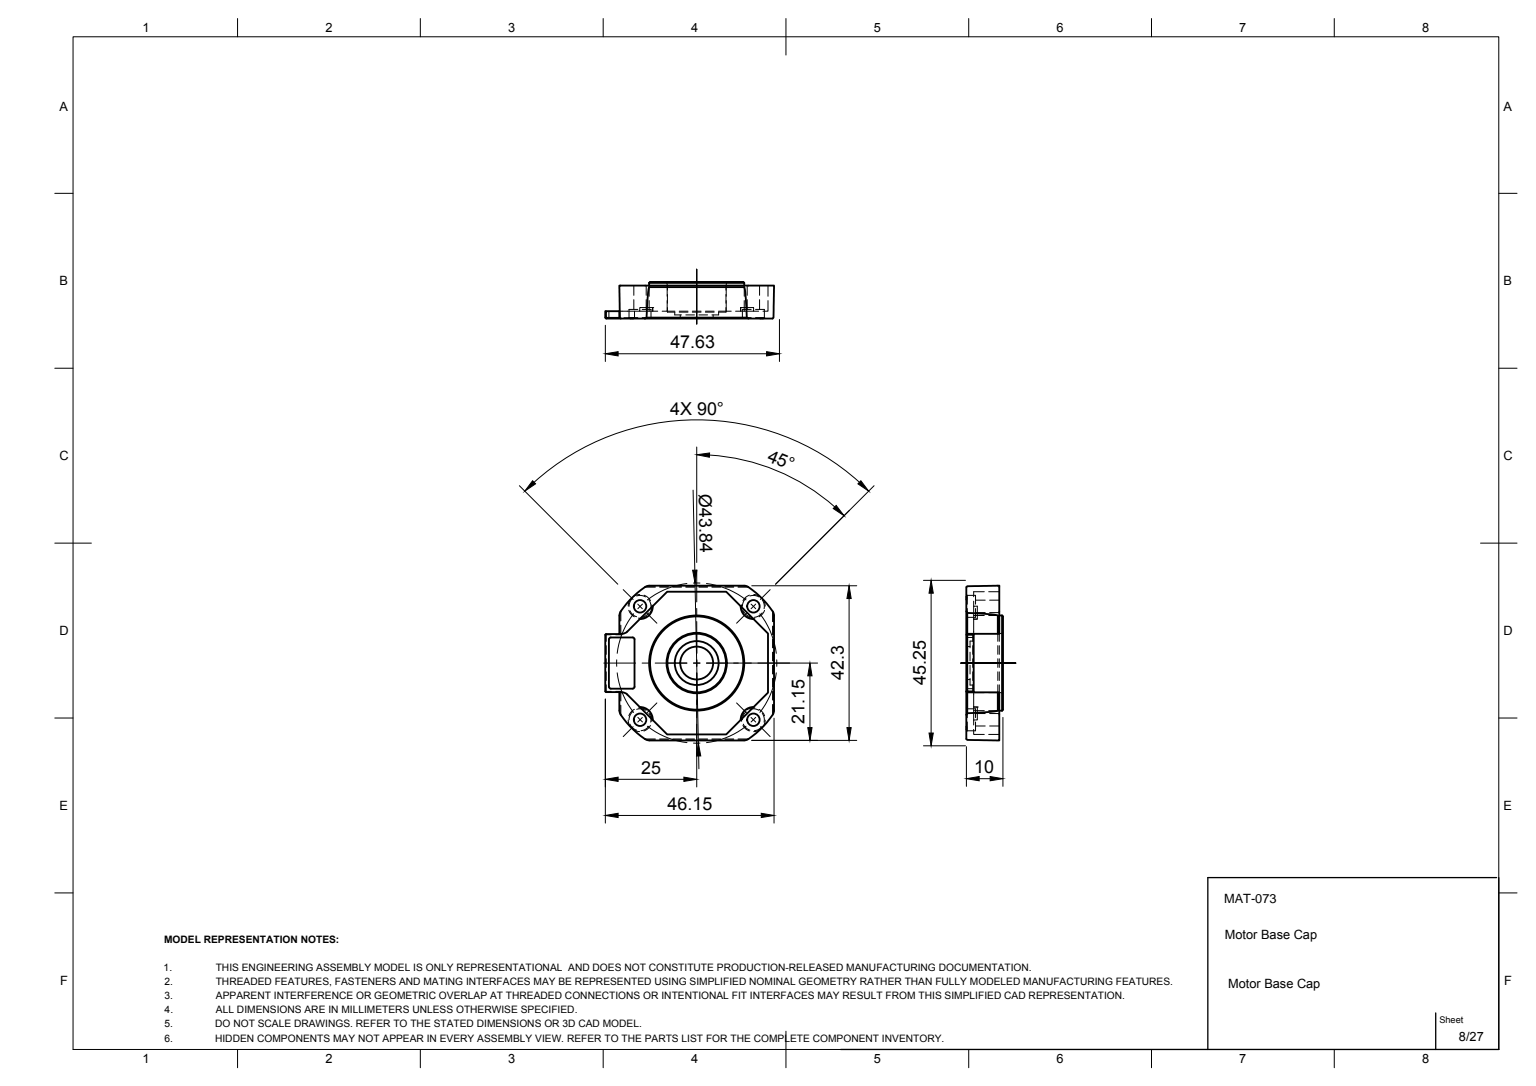
ISO-10303-21;
HEADER;
/* Generated by software containing ST-Developer
 * from STEP Tools, Inc. (www.steptools.com) 
 */

FILE_DESCRIPTION(
/* description */ ('CAx-IF Rec.Pracs.---Representation and Presentation of Product Manufa
cturing Information (PMI)---4.0---2014-10-13'),
/* implementation_level */ '2;1');

FILE_NAME(
/* name */ 'Motor Base Cap.step',
/* time_stamp */ '2026-10-24T18:52:33-07:00',
/* author */ (''),
/* organization */ (''),
/* preprocessor_version */ 'ST-DEVELOPER v20.2',
/* originating_system */ 'Autodesk Translation Framework v15.17.0.0',
/* authorisation */ '');

FILE_SCHEMA (('AP242_MANAGED_MODEL_BASED_3D_ENGINEERING_MIM_LF { 1 0 10303 442 2 1 4 }'));
ENDSEC;

DATA;
#10=MECHANICAL_DESIGN_GEOMETRIC_PRESENTATION_REPRESENTATION('',(#419),#34876);
#174=CONICAL_SURFACE('',#20658,0.003125,0.785398163397447);
#175=CONICAL_SURFACE('',#20665,0.003125,0.785398163397447);
#176=CONICAL_SURFACE('',#20672,0.003125,0.785398163397447);
#177=CONICAL_SURFACE('',#20689,0.003125,0.785398163397447);
#178=CONICAL_SURFACE('',#20758,0.012875,0.785398163397446);
#179=CONICAL_SURFACE('',#20765,0.008125,0.244978663126864);
#216=B_SPLINE_CURVE_WITH_KNOTS('',3,(#30332,#30333,#30334,#30335,#30336,
#30337),.UNSPECIFIED.,.F.,.F.,(4,2,4),(1.58777834959488,1.67090244580867,
1.70100758687363),.UNSPECIFIED.);
#217=B_SPLINE_CURVE_WITH_KNOTS('',3,(#30373,#30374,#30375,#30376,#30377,
#30378),.UNSPECIFIED.,.F.,.F.,(4,2,4),(1.58777834958732,1.67090244580931,
1.70100758688213),.UNSPECIFIED.);
#218=B_SPLINE_CURVE_WITH_KNOTS('',3,(#30414,#30415,#30416,#30417,#30418,
#30419),.UNSPECIFIED.,.F.,.F.,(4,2,4),(1.58777834957897,1.67090244581023,
1.70100758689154),.UNSPECIFIED.);
#219=B_SPLINE_CURVE_WITH_KNOTS('',3,(#30471,#30472,#30473,#30474,#30475,
#30476),.UNSPECIFIED.,.F.,.F.,(4,2,4),(1.58777834959617,1.67090244580851,
1.70100758687202),.UNSPECIFIED.);
#300=ELLIPSE('',#20594,0.114597376996511,0.00199999999998973);
#301=ELLIPSE('',#20596,0.00280406412973375,0.00199999999998973);
#302=ELLIPSE('',#20598,0.0352260556299788,0.0251250000000126);
#303=ELLIPSE('',#20600,0.0352260556299788,0.0251250000000126);
#304=ELLIPSE('',#20604,0.00280406412976774,0.00200000000001397);
#305=ELLIPSE('',#20606,0.114597376997899,0.00200000000001397);
#306=ELLIPSE('',#20609,0.114597376996524,0.00199999999998997);
#307=ELLIPSE('',#20611,0.00280406412973409,0.00199999999998997);
#308=ELLIPSE('',#20613,0.0352260556299805,0.0251250000000138);
#309=ELLIPSE('',#20615,0.0352260556299805,0.0251250000000138);
#310=ELLIPSE('',#20619,0.00280406412974482,0.00199999999999762);
#311=ELLIPSE('',#20621,0.114597376996964,0.00199999999999762);
#312=ELLIPSE('',#20624,0.114597376997842,0.00200000000001296);
#313=ELLIPSE('',#20626,0.00280406412976633,0.00200000000001296);
#314=ELLIPSE('',#20628,0.0352260556299806,0.0251250000000138);
#315=ELLIPSE('',#20630,0.0352260556299803,0.0251250000000138);
#316=ELLIPSE('',#20638,0.00280406412973409,0.00199999999998998);
#317=ELLIPSE('',#20639,0.114597376996526,0.00199999999998998);
#318=ELLIPSE('',#20642,0.0352260556300019,0.0251250000000291);
#319=ELLIPSE('',#20645,0.0352260556300016,0.0251250000000291);
#320=ELLIPSE('',#20648,0.114597376997269,0.00200000000000295);
#321=ELLIPSE('',#20649,0.00280406412975229,0.00200000000000295);
#322=ELLIPSE('',#20653,0.114597376996301,0.00199999999998605);
#323=ELLIPSE('',#20654,0.00280406412972858,0.00199999999998605);
#353=SHAPE_REPRESENTATION_RELATIONSHIP('SRR','None',#34990,#386);
#386=ADVANCED_BREP_SHAPE_REPRESENTATION('',(#452),#34848);
#419=STYLED_ITEM('',(#35159),#452);
#452=MANIFOLD_SOLID_BREP('Motor Base Cap',#19559);
#503=FACE_BOUND('',#6175,.T.);
#504=FACE_BOUND('',#6184,.T.);
#505=FACE_BOUND('',#6185,.T.);
#506=FACE_BOUND('',#6186,.T.);
#507=FACE_BOUND('',#6187,.T.);
#508=FACE_BOUND('',#6224,.T.);
#509=FACE_BOUND('',#6229,.T.);
#510=FACE_BOUND('',#6232,.T.);
#511=FACE_BOUND('',#6235,.T.);
#512=FACE_BOUND('',#6238,.T.);
#513=FACE_BOUND('',#6241,.T.);
#514=FACE_BOUND('',#6242,.T.);
#515=FACE_BOUND('',#6245,.T.);
#516=FACE_BOUND('',#6247,.T.);
#719=PLANE('',#20592);
#720=PLANE('',#20607);
#721=PLANE('',#20622);
#722=PLANE('',#20633);
#723=PLANE('',#20634);
#724=PLANE('',#20635);
#725=PLANE('',#20636);
#726=PLANE('',#20655);
#727=PLANE('',#20656);
#728=PLANE('',#20657);
#729=PLANE('',#20663);
#730=PLANE('',#20664);
#731=PLANE('',#20670);
#732=PLANE('',#20671);
#733=PLANE('',#20677);
#734=PLANE('',#20678);
#735=PLANE('',#20679);
#736=PLANE('',#20680);
#737=PLANE('',#20681);
#738=PLANE('',#20699);
#739=PLANE('',#20700);
#740=PLANE('',#20708);
#741=PLANE('',#20709);
#742=PLANE('',#20710);
#743=PLANE('',#20711);
#744=PLANE('',#20712);
#745=PLANE('',#20713);
#746=PLANE('',#20714);
#747=PLANE('',#20718);
#748=PLANE('',#20722);
#749=PLANE('',#20726);
#750=PLANE('',#20730);
#751=PLANE('',#20731);
#752=PLANE('',#20732);
#753=PLANE('',#20733);
#754=PLANE('',#20736);
#755=PLANE('',#20737);
#756=PLANE('',#20741);
#757=PLANE('',#20745);
#758=PLANE('',#20749);
#759=PLANE('',#20750);
#760=PLANE('',#20751);
#761=PLANE('',#20755);
#762=PLANE('',#20756);
#763=PLANE('',#20757);
#764=PLANE('',#20761);
#765=PLANE('',#20770);
#766=PLANE('',#20773);
#767=PLANE('',#20776);
#768=PLANE('',#20779);
#769=PLANE('',#20782);
#770=PLANE('',#20786);
#771=PLANE('',#20787);
#772=PLANE('',#20788);
#773=PLANE('',#20789);
#774=PLANE('',#20790);
#775=PLANE('',#20791);
#1478=LINE('',#30306,#3077);
#1479=LINE('',#30308,#3078);
#1480=LINE('',#30310,#3079);
#1481=LINE('',#30311,#3080);
#1482=LINE('',#30318,#3081);
#1483=LINE('',#30326,#3082);
#1484=LINE('',#30345,#3083);
#1485=LINE('',#30349,#3084);
#1486=LINE('',#30351,#3085);
#1487=LINE('',#30352,#3086);
#1488=LINE('',#30359,#3087);
#1489=LINE('',#30367,#3088);
#1490=LINE('',#30386,#3089);
#1491=LINE('',#30390,#3090);
#1492=LINE('',#30392,#3091);
#1493=LINE('',#30393,#3092);
#1494=LINE('',#30400,#3093);
#1495=LINE('',#30408,#3094);
#1496=LINE('',#30424,#3095);
#1497=LINE('',#30426,#3096);
#1498=LINE('',#30428,#3097);
#1499=LINE('',#30429,#3098);
#1500=LINE('',#30433,#3099);
#1501=LINE('',#30435,#3100);
#1502=LINE('',#30437,#3101);
#1503=LINE('',#30438,#3102);
#1504=LINE('',#30441,#3103);
#1505=LINE('',#30443,#3104);
#1506=LINE('',#30445,#3105);
#1507=LINE('',#30446,#3106);
#1508=LINE('',#30450,#3107);
#1509=LINE('',#30452,#3108);
#1510=LINE('',#30454,#3109);
#1511=LINE('',#30455,#3110);
#1512=LINE('',#30463,#3111);
#1513=LINE('',#30482,#3112);
#1514=LINE('',#30492,#3113);
#1515=LINE('',#30498,#3114);
#1516=LINE('',#30500,#3115);
#1517=LINE('',#30501,#3116);
#1518=LINE('',#30504,#3117);
#1519=LINE('',#30506,#3118);
#1520=LINE('',#30508,#3119);
#1521=LINE('',#30509,#3120);
#1522=LINE('',#30511,#3121);
#1523=LINE('',#30517,#3122);
#1524=LINE('',#30522,#3123);
#1525=LINE('',#30524,#3124);
#1526=LINE('',#30530,#3125);
#1527=LINE('',#30535,#3126);
#1528=LINE('',#30537,#3127);
#1529=LINE('',#30543,#3128);
#1530=LINE('',#30549,#3129);
#1531=LINE('',#30551,#3130);
#1532=LINE('',#30552,#3131);
#1533=LINE('',#30555,#3132);
#1534=LINE('',#30557,#3133);
#1535=LINE('',#30558,#3134);
#1536=LINE('',#30561,#3135);
#1537=LINE('',#30562,#3136);
#1538=LINE('',#30563,#3137);
#1539=LINE('',#30566,#3138);
#1540=LINE('',#30568,#3139);
#1541=LINE('',#30569,#3140);
#1542=LINE('',#30571,#3141);
#1543=LINE('',#30573,#3142);
#1544=LINE('',#30575,#3143);
#1545=LINE('',#30576,#3144);
#1546=LINE('',#30585,#3145);
#1547=LINE('',#30589,#3146);
#1548=LINE('',#30594,#3147);
#1549=LINE('',#30599,#3148);
#1550=LINE('',#30603,#3149);
#1551=LINE('',#30609,#3150);
#1552=LINE('',#30612,#3151);
#1553=LINE('',#30615,#3152);
#1554=LINE('',#30616,#3153);
#1555=LINE('',#30617,#3154);
#1556=LINE('',#30620,#3155);
#1557=LINE('',#30622,#3156);
#1558=LINE('',#30624,#3157);
#1559=LINE('',#30626,#3158);
#1560=LINE('',#30628,#3159);
#1561=LINE('',#30630,#3160);
#1562=LINE('',#30632,#3161);
#1563=LINE('',#30635,#3162);
#1564=LINE('',#30646,#3163);
#1565=LINE('',#30649,#3164);
#1566=LINE('',#30652,#3165);
#1567=LINE('',#30654,#3166);
#1568=LINE('',#30656,#3167);
#1569=LINE('',#30658,#3168);
#1570=LINE('',#30660,#3169);
#1571=LINE('',#30661,#3170);
#1572=LINE('',#30663,#3171);
#1573=LINE('',#30664,#3172);
#1574=LINE('',#30666,#3173);
#1575=LINE('',#30667,#3174);
#1576=LINE('',#30670,#3175);
#1577=LINE('',#30671,#3176);
#1578=LINE('',#30674,#3177);
#1579=LINE('',#30675,#3178);
#1580=LINE('',#30677,#3179);
#1581=LINE('',#30680,#3180);
#1582=LINE('',#30682,#3181);
#1583=LINE('',#30683,#3182);
#1584=LINE('',#30689,#3183);
#1585=LINE('',#30692,#3184);
#1586=LINE('',#30695,#3185);
#1587=LINE('',#30697,#3186);
#1588=LINE('',#30698,#3187);
#1589=LINE('',#30703,#3188);
#1590=LINE('',#30707,#3189);
#1591=LINE('',#30709,#3190);
#1592=LINE('',#30710,#3191);
#1593=LINE('',#30715,#3192);
#1594=LINE('',#30719,#3193);
#1595=LINE('',#30721,#3194);
#1596=LINE('',#30722,#3195);
#1597=LINE('',#30727,#3196);
#1598=LINE('',#30730,#3197);
#1599=LINE('',#30732,#3198);
#1600=LINE('',#30735,#3199);
#1601=LINE('',#30739,#3200);
#1602=LINE('',#30741,#3201);
#1603=LINE('',#30742,#3202);
#1604=LINE('',#30744,#3203);
#1605=LINE('',#30750,#3204);
#1606=LINE('',#30753,#3205);
#1607=LINE('',#30755,#3206);
#1608=LINE('',#30765,#3207);
#1609=LINE('',#30768,#3208);
#1610=LINE('',#30770,#3209);
#1611=LINE('',#30772,#3210);
#1612=LINE('',#30774,#3211);
#1613=LINE('',#30775,#3212);
#1614=LINE('',#30778,#3213);
#1615=LINE('',#30779,#3214);
#1616=LINE('',#30781,#3215);
#1617=LINE('',#30782,#3216);
#1618=LINE('',#30788,#3217);
#1619=LINE('',#30791,#3218);
#1620=LINE('',#30793,#3219);
#1621=LINE('',#30796,#3220);
#1622=LINE('',#30797,#3221);
#1623=LINE('',#30799,#3222);
#1624=LINE('',#30800,#3223);
#1625=LINE('',#30806,#3224);
#1626=LINE('',#30814,#3225);
#1627=LINE('',#30819,#3226);
#1628=LINE('',#30823,#3227);
#1629=LINE('',#30829,#3228);
#1630=LINE('',#30834,#3229);
#1631=LINE('',#30839,#3230);
#1632=LINE('',#30844,#3231);
#1633=LINE('',#30846,#3232);
#1634=LINE('',#30847,#3233);
#1635=LINE('',#30848,#3234);
#1636=LINE('',#30853,#3235);
#3077=VECTOR('',#23937,0.01);
#3078=VECTOR('',#23938,0.01);
#3079=VECTOR('',#23939,0.01);
#3080=VECTOR('',#23940,0.01);
#3081=VECTOR('',#23947,0.01);
#3082=VECTOR('',#23956,0.01);
#3083=VECTOR('',#23969,0.01);
#3084=VECTOR('',#23974,0.01);
#3085=VECTOR('',#23975,0.01);
#3086=VECTOR('',#23976,0.01);
#3087=VECTOR('',#23983,0.01);
#3088=VECTOR('',#23992,0.01);
#3089=VECTOR('',#24005,0.01);
#3090=VECTOR('',#24010,0.01);
#3091=VECTOR('',#24011,0.01);
#3092=VECTOR('',#24012,0.01);
#3093=VECTOR('',#24019,0.01);
#3094=VECTOR('',#24028,0.01);
#3095=VECTOR('',#24037,0.01);
#3096=VECTOR('',#24038,0.01);
#3097=VECTOR('',#24039,0.01);
#3098=VECTOR('',#24040,0.01);
#3099=VECTOR('',#24043,0.01);
#3100=VECTOR('',#24044,0.01);
#3101=VECTOR('',#24045,0.01);
#3102=VECTOR('',#24046,0.01);
#3103=VECTOR('',#24049,0.01);
#3104=VECTOR('',#24050,0.01);
#3105=VECTOR('',#24051,0.01);
#3106=VECTOR('',#24052,0.01);
#3107=VECTOR('',#24055,0.01);
#3108=VECTOR('',#24056,0.01);
#3109=VECTOR('',#24057,0.01);
#3110=VECTOR('',#24058,0.01);
#3111=VECTOR('',#24067,0.01);
#3112=VECTOR('',#24080,0.01);
#3113=VECTOR('',#24093,0.01);
#3114=VECTOR('',#24100,0.01);
#3115=VECTOR('',#24101,0.01);
#3116=VECTOR('',#24102,0.01);
#3117=VECTOR('',#24105,0.01);
#3118=VECTOR('',#24106,0.01);
#3119=VECTOR('',#24107,0.01);
#3120=VECTOR('',#24108,0.01);
#3121=VECTOR('',#24111,1.);
#3122=VECTOR('',#24116,0.003125);
#3123=VECTOR('',#24125,1.);
#3124=VECTOR('',#24128,1.);
#3125=VECTOR('',#24133,0.003125);
#3126=VECTOR('',#24142,1.);
#3127=VECTOR('',#24145,1.);
#3128=VECTOR('',#24150,0.003125);
#3129=VECTOR('',#24159,1.);
#3130=VECTOR('',#24160,1.);
#3131=VECTOR('',#24161,1.);
#3132=VECTOR('',#24164,1.);
#3133=VECTOR('',#24165,1.);
#3134=VECTOR('',#24166,1.);
#3135=VECTOR('',#24169,1.);
#3136=VECTOR('',#24170,1.);
#3137=VECTOR('',#24171,1.);
#3138=VECTOR('',#24174,1.);
#3139=VECTOR('',#24175,1.);
#3140=VECTOR('',#24176,1.);
#3141=VECTOR('',#24179,1.);
#3142=VECTOR('',#24180,1.);
#3143=VECTOR('',#24181,1.);
#3144=VECTOR('',#24182,1.);
#3145=VECTOR('',#24193,0.003);
#3146=VECTOR('',#24198,0.003);
#3147=VECTOR('',#24203,0.003125);
#3148=VECTOR('',#24210,0.003);
#3149=VECTOR('',#24215,0.003);
#3150=VECTOR('',#24220,1.);
#3151=VECTOR('',#24223,1.);
#3152=VECTOR('',#24226,1.);
#3153=VECTOR('',#24227,1.);
#3154=VECTOR('',#24228,1.);
#3155=VECTOR('',#24231,1.);
#3156=VECTOR('',#24232,1.);
#3157=VECTOR('',#24233,1.);
#3158=VECTOR('',#24234,1.);
#3159=VECTOR('',#24235,1.);
#3160=VECTOR('',#24236,1.);
#3161=VECTOR('',#24237,1.);
#3162=VECTOR('',#24240,1.);
#3163=VECTOR('',#24251,1.);
#3164=VECTOR('',#24254,1.);
#3165=VECTOR('',#24257,1.);
#3166=VECTOR('',#24258,1.);
#3167=VECTOR('',#24259,1.);
#3168=VECTOR('',#24260,1.);
#3169=VECTOR('',#24261,1.);
#3170=VECTOR('',#24262,1.);
#3171=VECTOR('',#24265,1.);
#3172=VECTOR('',#24266,1.);
#3173=VECTOR('',#24269,1.);
#3174=VECTOR('',#24270,1.);
#3175=VECTOR('',#24273,1.);
#3176=VECTOR('',#24274,1.);
#3177=VECTOR('',#24277,1.);
#3178=VECTOR('',#24278,1.);
#3179=VECTOR('',#24281,1.);
#3180=VECTOR('',#24284,1.);
#3181=VECTOR('',#24285,1.);
#3182=VECTOR('',#24286,1.);
#3183=VECTOR('',#24291,1.);
#3184=VECTOR('',#24294,1.);
#3185=VECTOR('',#24297,1.);
#3186=VECTOR('',#24298,1.);
#3187=VECTOR('',#24299,1.);
#3188=VECTOR('',#24304,1.);
#3189=VECTOR('',#24309,1.);
#3190=VECTOR('',#24310,1.);
#3191=VECTOR('',#24311,1.);
#3192=VECTOR('',#24316,1.);
#3193=VECTOR('',#24321,1.);
#3194=VECTOR('',#24322,1.);
#3195=VECTOR('',#24323,1.);
#3196=VECTOR('',#24328,1.);
#3197=VECTOR('',#24333,1.);
#3198=VECTOR('',#24336,1.);
#3199=VECTOR('',#24341,1.);
#3200=VECTOR('',#24346,0.0045);
#3201=VECTOR('',#24349,1.);
#3202=VECTOR('',#24350,1.);
#3203=VECTOR('',#24353,1.);
#3204=VECTOR('',#24358,1.);
#3205=VECTOR('',#24361,1.);
#3206=VECTOR('',#24364,1.);
#3207=VECTOR('',#24377,1.);
#3208=VECTOR('',#24380,1.);
#3209=VECTOR('',#24383,1.);
#3210=VECTOR('',#24386,1.);
#3211=VECTOR('',#24387,1.);
#3212=VECTOR('',#24388,1.);
#3213=VECTOR('',#24391,1.);
#3214=VECTOR('',#24392,1.);
#3215=VECTOR('',#24393,1.);
#3216=VECTOR('',#24394,1.);
#3217=VECTOR('',#24399,1.);
#3218=VECTOR('',#24402,1.);
#3219=VECTOR('',#24405,1.);
#3220=VECTOR('',#24408,1.);
#3221=VECTOR('',#24409,1.);
#3222=VECTOR('',#24410,1.);
#3223=VECTOR('',#24411,1.);
#3224=VECTOR('',#24418,0.012875);
#3225=VECTOR('',#24429,0.013);
#3226=VECTOR('',#24434,0.008125);
#3227=VECTOR('',#24439,0.008);
#3228=VECTOR('',#24448,0.0017);
#3229=VECTOR('',#24455,0.0017);
#3230=VECTOR('',#24462,0.0017);
#3231=VECTOR('',#24469,0.0017);
#3232=VECTOR('',#24472,1.);
#3233=VECTOR('',#24473,1.);
#3234=VECTOR('',#24474,1.);
#3235=VECTOR('',#24479,0.006);
#4430=CYLINDRICAL_SURFACE('',#20593,0.00199999999998973);
#4431=CYLINDRICAL_SURFACE('',#20597,0.0251250000000126);
#4432=CYLINDRICAL_SURFACE('',#20603,0.00200000000001397);
#4433=CYLINDRICAL_SURFACE('',#20608,0.00199999999998997);
#4434=CYLINDRICAL_SURFACE('',#20612,0.0251250000000138);
#4435=CYLINDRICAL_SURFACE('',#20618,0.00199999999999762);
#4436=CYLINDRICAL_SURFACE('',#20623,0.00200000000001296);
#4437=CYLINDRICAL_SURFACE('',#20627,0.0251250000000138);
#4438=CYLINDRICAL_SURFACE('',#20637,0.00199999999998998);
#4439=CYLINDRICAL_SURFACE('',#20641,0.0251250000000291);
#4440=CYLINDRICAL_SURFACE('',#20647,0.00200000000000295);
#4441=CYLINDRICAL_SURFACE('',#20651,0.00199999999998605);
#4442=CYLINDRICAL_SURFACE('',#20685,0.003);
#4443=CYLINDRICAL_SURFACE('',#20687,0.003);
#4444=CYLINDRICAL_SURFACE('',#20692,0.003);
#4445=CYLINDRICAL_SURFACE('',#20694,0.003);
#4446=CYLINDRICAL_SURFACE('',#20696,0.002);
#4447=CYLINDRICAL_SURFACE('',#20706,0.002);
#4448=CYLINDRICAL_SURFACE('',#20715,0.0005);
#4449=CYLINDRICAL_SURFACE('',#20719,0.0005);
#4450=CYLINDRICAL_SURFACE('',#20723,0.0005);
#4451=CYLINDRICAL_SURFACE('',#20727,0.0005);
#4452=CYLINDRICAL_SURFACE('',#20734,0.0045);
#4453=CYLINDRICAL_SURFACE('',#20738,0.00347964100813058);
#4454=CYLINDRICAL_SURFACE('',#20742,0.00347964100813058);
#4455=CYLINDRICAL_SURFACE('',#20746,0.00347964100813058);
#4456=CYLINDRICAL_SURFACE('',#20752,0.00347964100813058);
#4457=CYLINDRICAL_SURFACE('',#20763,0.013);
#4458=CYLINDRICAL_SURFACE('',#20768,0.008);
#4459=CYLINDRICAL_SURFACE('',#20772,0.0017);
#4460=CYLINDRICAL_SURFACE('',#20775,0.0017);
#4461=CYLINDRICAL_SURFACE('',#20778,0.0017);
#4462=CYLINDRICAL_SURFACE('',#20781,0.0017);
#4463=CYLINDRICAL_SURFACE('',#20783,0.006);
#5073=FACE_OUTER_BOUND('',#6141,.T.);
#5074=FACE_OUTER_BOUND('',#6142,.T.);
#5075=FACE_OUTER_BOUND('',#6143,.T.);
#5076=FACE_OUTER_BOUND('',#6144,.T.);
#5077=FACE_OUTER_BOUND('',#6145,.T.);
#5078=FACE_OUTER_BOUND('',#6146,.T.);
#5079=FACE_OUTER_BOUND('',#6147,.T.);
#5080=FACE_OUTER_BOUND('',#6148,.T.);
#5081=FACE_OUTER_BOUND('',#6149,.T.);
#5082=FACE_OUTER_BOUND('',#6150,.T.);
#5083=FACE_OUTER_BOUND('',#6151,.T.);
#5084=FACE_OUTER_BOUND('',#6152,.T.);
#5085=FACE_OUTER_BOUND('',#6153,.T.);
#5086=FACE_OUTER_BOUND('',#6154,.T.);
#5087=FACE_OUTER_BOUND('',#6155,.T.);
#5088=FACE_OUTER_BOUND('',#6156,.T.);
#5089=FACE_OUTER_BOUND('',#6157,.T.);
#5090=FACE_OUTER_BOUND('',#6158,.T.);
#5091=FACE_OUTER_BOUND('',#6159,.T.);
#5092=FACE_OUTER_BOUND('',#6160,.T.);
#5093=FACE_OUTER_BOUND('',#6161,.T.);
#5094=FACE_OUTER_BOUND('',#6162,.T.);
#5095=FACE_OUTER_BOUND('',#6163,.T.);
#5096=FACE_OUTER_BOUND('',#6164,.T.);
#5097=FACE_OUTER_BOUND('',#6165,.T.);
#5098=FACE_OUTER_BOUND('',#6166,.T.);
#5099=FACE_OUTER_BOUND('',#6167,.T.);
#5100=FACE_OUTER_BOUND('',#6168,.T.);
#5101=FACE_OUTER_BOUND('',#6169,.T.);
#5102=FACE_OUTER_BOUND('',#6170,.T.);
#5103=FACE_OUTER_BOUND('',#6171,.T.);
#5104=FACE_OUTER_BOUND('',#6172,.T.);
#5105=FACE_OUTER_BOUND('',#6173,.T.);
#5106=FACE_OUTER_BOUND('',#6174,.T.);
#5107=FACE_OUTER_BOUND('',#6176,.T.);
#5108=FACE_OUTER_BOUND('',#6177,.T.);
#5109=FACE_OUTER_BOUND('',#6178,.T.);
#5110=FACE_OUTER_BOUND('',#6179,.T.);
#5111=FACE_OUTER_BOUND('',#6180,.T.);
#5112=FACE_OUTER_BOUND('',#6181,.T.);
#5113=FACE_OUTER_BOUND('',#6182,.T.);
#5114=FACE_OUTER_BOUND('',#6183,.T.);
#5115=FACE_OUTER_BOUND('',#6188,.T.);
#5116=FACE_OUTER_BOUND('',#6189,.T.);
#5117=FACE_OUTER_BOUND('',#6190,.T.);
#5118=FACE_OUTER_BOUND('',#6191,.T.);
#5119=FACE_OUTER_BOUND('',#6192,.T.);
#5120=FACE_OUTER_BOUND('',#6193,.T.);
#5121=FACE_OUTER_BOUND('',#6194,.T.);
#5122=FACE_OUTER_BOUND('',#6195,.T.);
#5123=FACE_OUTER_BOUND('',#6196,.T.);
#5124=FACE_OUTER_BOUND('',#6197,.T.);
#5125=FACE_OUTER_BOUND('',#6198,.T.);
#5126=FACE_OUTER_BOUND('',#6199,.T.);
#5127=FACE_OUTER_BOUND('',#6200,.T.);
#5128=FACE_OUTER_BOUND('',#6201,.T.);
#5129=FACE_OUTER_BOUND('',#6202,.T.);
#5130=FACE_OUTER_BOUND('',#6203,.T.);
#5131=FACE_OUTER_BOUND('',#6204,.T.);
#5132=FACE_OUTER_BOUND('',#6205,.T.);
#5133=FACE_OUTER_BOUND('',#6206,.T.);
#5134=FACE_OUTER_BOUND('',#6207,.T.);
#5135=FACE_OUTER_BOUND('',#6208,.T.);
#5136=FACE_OUTER_BOUND('',#6209,.T.);
#5137=FACE_OUTER_BOUND('',#6210,.T.);
#5138=FACE_OUTER_BOUND('',#6211,.T.);
#5139=FACE_OUTER_BOUND('',#6212,.T.);
#5140=FACE_OUTER_BOUND('',#6213,.T.);
#5141=FACE_OUTER_BOUND('',#6214,.T.);
#5142=FACE_OUTER_BOUND('',#6215,.T.);
#5143=FACE_OUTER_BOUND('',#6216,.T.);
#5144=FACE_OUTER_BOUND('',#6217,.T.);
#5145=FACE_OUTER_BOUND('',#6218,.T.);
#5146=FACE_OUTER_BOUND('',#6219,.T.);
#5147=FACE_OUTER_BOUND('',#6220,.T.);
#5148=FACE_OUTER_BOUND('',#6221,.T.);
#5149=FACE_OUTER_BOUND('',#6222,.T.);
#5150=FACE_OUTER_BOUND('',#6223,.T.);
#5151=FACE_OUTER_BOUND('',#6225,.T.);
#5152=FACE_OUTER_BOUND('',#6226,.T.);
#5153=FACE_OUTER_BOUND('',#6227,.T.);
#5154=FACE_OUTER_BOUND('',#6228,.T.);
#5155=FACE_OUTER_BOUND('',#6230,.T.);
#5156=FACE_OUTER_BOUND('',#6231,.T.);
#5157=FACE_OUTER_BOUND('',#6233,.T.);
#5158=FACE_OUTER_BOUND('',#6234,.T.);
#5159=FACE_OUTER_BOUND('',#6236,.T.);
#5160=FACE_OUTER_BOUND('',#6237,.T.);
#5161=FACE_OUTER_BOUND('',#6239,.T.);
#5162=FACE_OUTER_BOUND('',#6240,.T.);
#5163=FACE_OUTER_BOUND('',#6243,.T.);
#5164=FACE_OUTER_BOUND('',#6244,.T.);
#5165=FACE_OUTER_BOUND('',#6246,.T.);
#5166=FACE_OUTER_BOUND('',#6248,.T.);
#5167=FACE_OUTER_BOUND('',#6249,.T.);
#5168=FACE_OUTER_BOUND('',#6250,.T.);
#5169=FACE_OUTER_BOUND('',#6251,.T.);
#6141=EDGE_LOOP('',(#14336,#14337,#14338,#14339));
#6142=EDGE_LOOP('',(#14340,#14341,#14342,#14343,#14344));
#6143=EDGE_LOOP('',(#14345,#14346,#14347,#14348,#14349,#14350,#14351,#14352));
#6144=EDGE_LOOP('',(#14353,#14354,#14355,#14356,#14357));
#6145=EDGE_LOOP('',(#14358,#14359,#14360,#14361));
#6146=EDGE_LOOP('',(#14362,#14363,#14364,#14365,#14366));
#6147=EDGE_LOOP('',(#14367,#14368,#14369,#14370,#14371,#14372,#14373,#14374));
#6148=EDGE_LOOP('',(#14375,#14376,#14377,#14378,#14379));
#6149=EDGE_LOOP('',(#14380,#14381,#14382,#14383));
#6150=EDGE_LOOP('',(#14384,#14385,#14386,#14387,#14388));
#6151=EDGE_LOOP('',(#14389,#14390,#14391,#14392,#14393,#14394,#14395,#14396));
#6152=EDGE_LOOP('',(#14397,#14398,#14399,#14400));
#6153=EDGE_LOOP('',(#14401,#14402,#14403,#14404));
#6154=EDGE_LOOP('',(#14405,#14406,#14407,#14408,#14409));
#6155=EDGE_LOOP('',(#14410,#14411,#14412,#14413));
#6156=EDGE_LOOP('',(#14414,#14415,#14416,#14417,#14418));
#6157=EDGE_LOOP('',(#14419,#14420,#14421,#14422,#14423,#14424,#14425,#14426));
#6158=EDGE_LOOP('',(#14427,#14428,#14429,#14430,#14431));
#6159=EDGE_LOOP('',(#14432,#14433,#14434,#14435,#14436));
#6160=EDGE_LOOP('',(#14437,#14438,#14439,#14440));
#6161=EDGE_LOOP('',(#14441,#14442,#14443,#14444,#14445));
#6162=EDGE_LOOP('',(#14446,#14447,#14448,#14449));
#6163=EDGE_LOOP('',(#14450,#14451,#14452,#14453,#14454,#14455,#14456));
#6164=EDGE_LOOP('',(#14457,#14458,#14459,#14460));
#6165=EDGE_LOOP('',(#14461,#14462,#14463,#14464,#14465,#14466));
#6166=EDGE_LOOP('',(#14467,#14468,#14469,#14470,#14471,#14472,#14473));
#6167=EDGE_LOOP('',(#14474,#14475,#14476,#14477));
#6168=EDGE_LOOP('',(#14478,#14479,#14480,#14481,#14482,#14483));
#6169=EDGE_LOOP('',(#14484,#14485,#14486,#14487,#14488,#14489,#14490));
#6170=EDGE_LOOP('',(#14491,#14492,#14493,#14494,#14495));
#6171=EDGE_LOOP('',(#14496,#14497,#14498,#14499));
#6172=EDGE_LOOP('',(#14500,#14501,#14502,#14503,#14504,#14505,#14506));
#6173=EDGE_LOOP('',(#14507,#14508,#14509,#14510));
#6174=EDGE_LOOP('',(#14511,#14512,#14513,#14514,#14515,#14516,#14517,#14518,
#14519,#14520,#14521,#14522,#14523,#14524,#14525,#14526,#14527,#14528,#14529,
#14530,#14531,#14532,#14533,#14534));
#6175=EDGE_LOOP('',(#14535));
#6176=EDGE_LOOP('',(#14536,#14537,#14538,#14539,#14540));
#6177=EDGE_LOOP('',(#14541,#14542,#14543,#14544,#14545));
#6178=EDGE_LOOP('',(#14546,#14547,#14548,#14549,#14550,#14551,#14552));
#6179=EDGE_LOOP('',(#14553,#14554,#14555,#14556,#14557));
#6180=EDGE_LOOP('',(#14558,#14559,#14560,#14561,#14562));
#6181=EDGE_LOOP('',(#14563,#14564,#14565,#14566));
#6182=EDGE_LOOP('',(#14567,#14568,#14569,#14570,#14571));
#6183=EDGE_LOOP('',(#14572,#14573,#14574,#14575,#14576,#14577,#14578,#14579,
#14580,#14581,#14582,#14583,#14584,#14585,#14586,#14587,#14588,#14589,#14590,
#14591,#14592,#14593,#14594,#14595,#14596,#14597,#14598,#14599));
#6184=EDGE_LOOP('',(#14600));
#6185=EDGE_LOOP('',(#14601));
#6186=EDGE_LOOP('',(#14602));
#6187=EDGE_LOOP('',(#14603));
#6188=EDGE_LOOP('',(#14604,#14605,#14606,#14607));
#6189=EDGE_LOOP('',(#14608,#14609,#14610,#14611,#14612,#14613,#14614,#14615));
#6190=EDGE_LOOP('',(#14616,#14617,#14618,#14619,#14620));
#6191=EDGE_LOOP('',(#14621,#14622,#14623,#14624));
#6192=EDGE_LOOP('',(#14625,#14626,#14627,#14628));
#6193=EDGE_LOOP('',(#14629,#14630,#14631,#14632));
#6194=EDGE_LOOP('',(#14633,#14634,#14635,#14636));
#6195=EDGE_LOOP('',(#14637,#14638,#14639,#14640,#14641,#14642,#14643));
#6196=EDGE_LOOP('',(#14644,#14645,#14646,#14647));
#6197=EDGE_LOOP('',(#14648,#14649,#14650,#14651));
#6198=EDGE_LOOP('',(#14652,#14653,#14654,#14655));
#6199=EDGE_LOOP('',(#14656,#14657,#14658,#14659));
#6200=EDGE_LOOP('',(#14660,#14661,#14662,#14663));
#6201=EDGE_LOOP('',(#14664,#14665,#14666,#14667));
#6202=EDGE_LOOP('',(#14668,#14669,#14670,#14671));
#6203=EDGE_LOOP('',(#14672,#14673,#14674,#14675,#14676,#14677,#14678,#14679));
#6204=EDGE_LOOP('',(#14680,#14681,#14682,#14683));
#6205=EDGE_LOOP('',(#14684,#14685,#14686,#14687,#14688,#14689));
#6206=EDGE_LOOP('',(#14690,#14691,#14692,#14693,#14694));
#6207=EDGE_LOOP('',(#14695,#14696,#14697,#14698));
#6208=EDGE_LOOP('',(#14699,#14700,#14701,#14702));
#6209=EDGE_LOOP('',(#14703,#14704,#14705,#14706));
#6210=EDGE_LOOP('',(#14707,#14708,#14709,#14710));
#6211=EDGE_LOOP('',(#14711,#14712));
#6212=EDGE_LOOP('',(#14713,#14714,#14715,#14716));
#6213=EDGE_LOOP('',(#14717,#14718));
#6214=EDGE_LOOP('',(#14719,#14720,#14721,#14722));
#6215=EDGE_LOOP('',(#14723,#14724));
#6216=EDGE_LOOP('',(#14725,#14726,#14727,#14728,#14729,#14730,#14731,#14732));
#6217=EDGE_LOOP('',(#14733,#14734,#14735,#14736,#14737,#14738,#14739,#14740));
#6218=EDGE_LOOP('',(#14741,#14742,#14743,#14744));
#6219=EDGE_LOOP('',(#14745,#14746));
#6220=EDGE_LOOP('',(#14747,#14748,#14749,#14750,#14751,#14752,#14753,#14754));
#6221=EDGE_LOOP('',(#14755,#14756,#14757,#14758,#14759,#14760));
#6222=EDGE_LOOP('',(#14761,#14762,#14763,#14764));
#6223=EDGE_LOOP('',(#14765));
#6224=EDGE_LOOP('',(#14766));
#6225=EDGE_LOOP('',(#14767,#14768,#14769,#14770));
#6226=EDGE_LOOP('',(#14771,#14772,#14773,#14774,#14775));
#6227=EDGE_LOOP('',(#14776,#14777,#14778,#14779,#14780));
#6228=EDGE_LOOP('',(#14781));
#6229=EDGE_LOOP('',(#14782));
#6230=EDGE_LOOP('',(#14783,#14784,#14785,#14786));
#6231=EDGE_LOOP('',(#14787));
#6232=EDGE_LOOP('',(#14788));
#6233=EDGE_LOOP('',(#14789,#14790,#14791,#14792));
#6234=EDGE_LOOP('',(#14793));
#6235=EDGE_LOOP('',(#14794));
#6236=EDGE_LOOP('',(#14795,#14796,#14797,#14798));
#6237=EDGE_LOOP('',(#14799));
#6238=EDGE_LOOP('',(#14800));
#6239=EDGE_LOOP('',(#14801,#14802,#14803,#14804));
#6240=EDGE_LOOP('',(#14805,#14806,#14807,#14808,#14809,#14810,#14811,#14812,
#14813,#14814,#14815,#14816,#14817,#14818,#14819,#14820,#14821,#14822,#14823,
#14824,#14825,#14826,#14827,#14828,#14829,#14830,#14831,#14832));
#6241=EDGE_LOOP('',(#14833,#14834,#14835,#14836,#14837,#14838,#14839,#14840));
#6242=EDGE_LOOP('',(#14841));
#6243=EDGE_LOOP('',(#14842,#14843,#14844,#14845));
#6244=EDGE_LOOP('',(#14846));
#6245=EDGE_LOOP('',(#14847));
#6246=EDGE_LOOP('',(#14848));
#6247=EDGE_LOOP('',(#14849));
#6248=EDGE_LOOP('',(#14850,#14851,#14852,#14853));
#6249=EDGE_LOOP('',(#14854,#14855,#14856,#14857));
#6250=EDGE_LOOP('',(#14858,#14859,#14860,#14861));
#6251=EDGE_LOOP('',(#14862,#14863,#14864,#14865,#14866,#14867));
#7283=CIRCLE('',#20595,0.00199999999998973);
#7284=CIRCLE('',#20599,0.0251250000000126);
#7285=CIRCLE('',#20601,0.0251250000000126);
#7286=CIRCLE('',#20602,0.0251250000000126);
#7287=CIRCLE('',#20605,0.00200000000001397);
#7288=CIRCLE('',#20610,0.00199999999998997);
#7289=CIRCLE('',#20614,0.0251250000000138);
#7290=CIRCLE('',#20616,0.0251250000000138);
#7291=CIRCLE('',#20617,0.0251250000000138);
#7292=CIRCLE('',#20620,0.00199999999999762);
#7293=CIRCLE('',#20625,0.00200000000001296);
#7294=CIRCLE('',#20629,0.0251250000000138);
#7295=CIRCLE('',#20631,0.0251250000000138);
#7296=CIRCLE('',#20632,0.0251250000000138);
#7297=CIRCLE('',#20640,0.00199999999998998);
#7298=CIRCLE('',#20643,0.0251250000000291);
#7299=CIRCLE('',#20644,0.0251250000000291);
#7300=CIRCLE('',#20646,0.0251250000000291);
#7301=CIRCLE('',#20650,0.00200000000000295);
#7302=CIRCLE('',#20652,0.00199999999998605);
#7303=CIRCLE('',#20659,0.00300000000001);
#7304=CIRCLE('',#20660,0.00325000000001);
#7305=CIRCLE('',#20661,0.00325000000001);
#7306=CIRCLE('',#20662,0.00300000000001);
#7307=CIRCLE('',#20666,0.00300000000001);
#7308=CIRCLE('',#20667,0.00325000000001);
#7309=CIRCLE('',#20668,0.00325000000001);
#7310=CIRCLE('',#20669,0.00300000000001);
#7311=CIRCLE('',#20673,0.00300000000001);
#7312=CIRCLE('',#20674,0.00325000000001);
#7313=CIRCLE('',#20675,0.00325000000001);
#7314=CIRCLE('',#20676,0.00300000000001);
#7315=CIRCLE('',#20682,0.00325000000001);
#7316=CIRCLE('',#20683,0.00325000000001);
#7317=CIRCLE('',#20684,0.00450000000001);
#7318=CIRCLE('',#20686,0.00300000000001);
#7319=CIRCLE('',#20688,0.00300000000001);
#7320=CIRCLE('',#20690,0.00300000000001);
#7321=CIRCLE('',#20691,0.00300000000001);
#7322=CIRCLE('',#20693,0.00300000000001);
#7323=CIRCLE('',#20695,0.00300000000001);
#7324=CIRCLE('',#20697,0.00200000000001414);
#7325=CIRCLE('',#20698,0.00200000000001414);
#7326=CIRCLE('',#20701,0.00200000000001);
#7327=CIRCLE('',#20702,0.00170000000001);
#7328=CIRCLE('',#20703,0.00170000000001);
#7329=CIRCLE('',#20704,0.00170000000001);
#7330=CIRCLE('',#20705,0.00170000000001);
#7331=CIRCLE('',#20707,0.00200000000001);
#7332=CIRCLE('',#20716,0.000500000000014142);
#7333=CIRCLE('',#20717,0.000500000000014142);
#7334=CIRCLE('',#20720,0.000500000000014142);
#7335=CIRCLE('',#20721,0.000500000000014142);
#7336=CIRCLE('',#20724,0.000500000000014142);
#7337=CIRCLE('',#20725,0.000500000000014142);
#7338=CIRCLE('',#20728,0.000500000000014142);
#7339=CIRCLE('',#20729,0.000500000000014142);
#7340=CIRCLE('',#20735,0.00450000000001);
#7341=CIRCLE('',#20739,0.00347964100814074);
#7342=CIRCLE('',#20740,0.00347964100814074);
#7343=CIRCLE('',#20743,0.00347964100814074);
#7344=CIRCLE('',#20744,0.00347964100814074);
#7345=CIRCLE('',#20747,0.00347964100814074);
#7346=CIRCLE('',#20748,0.00347964100814074);
#7347=CIRCLE('',#20753,0.00347964100814074);
#7348=CIRCLE('',#20754,0.00347964100814074);
#7349=CIRCLE('',#20759,0.01300000000001);
#7350=CIRCLE('',#20760,0.01275000000001);
#7351=CIRCLE('',#20762,0.00825000000001);
#7352=CIRCLE('',#20764,0.01300000000001);
#7353=CIRCLE('',#20766,0.00800000000001);
#7354=CIRCLE('',#20767,0.00800000000001);
#7355=CIRCLE('',#20769,0.00800000000001);
#7356=CIRCLE('',#20771,0.00170000000001);
#7357=CIRCLE('',#20774,0.00170000000001);
#7358=CIRCLE('',#20777,0.00170000000001);
#7359=CIRCLE('',#20780,0.00170000000001);
#7360=CIRCLE('',#20784,0.00600000000001);
#7361=CIRCLE('',#20785,0.00600000000001);
#8581=VERTEX_POINT('',#30304);
#8582=VERTEX_POINT('',#30305);
#8583=VERTEX_POINT('',#30307);
#8584=VERTEX_POINT('',#30309);
#8585=VERTEX_POINT('',#30313);
#8586=VERTEX_POINT('',#30315);
#8587=VERTEX_POINT('',#30317);
#8588=VERTEX_POINT('',#30321);
#8589=VERTEX_POINT('',#30323);
#8590=VERTEX_POINT('',#30325);
#8591=VERTEX_POINT('',#30327);
#8592=VERTEX_POINT('',#30329);
#8593=VERTEX_POINT('',#30331);
#8594=VERTEX_POINT('',#30340);
#8595=VERTEX_POINT('',#30342);
#8596=VERTEX_POINT('',#30344);
#8597=VERTEX_POINT('',#30348);
#8598=VERTEX_POINT('',#30350);
#8599=VERTEX_POINT('',#30354);
#8600=VERTEX_POINT('',#30356);
#8601=VERTEX_POINT('',#30358);
#8602=VERTEX_POINT('',#30362);
#8603=VERTEX_POINT('',#30364);
#8604=VERTEX_POINT('',#30366);
#8605=VERTEX_POINT('',#30368);
#8606=VERTEX_POINT('',#30370);
#8607=VERTEX_POINT('',#30372);
#8608=VERTEX_POINT('',#30381);
#8609=VERTEX_POINT('',#30383);
#8610=VERTEX_POINT('',#30385);
#8611=VERTEX_POINT('',#30389);
#8612=VERTEX_POINT('',#30391);
#8613=VERTEX_POINT('',#30395);
#8614=VERTEX_POINT('',#30397);
#8615=VERTEX_POINT('',#30399);
#8616=VERTEX_POINT('',#30403);
#8617=VERTEX_POINT('',#30405);
#8618=VERTEX_POINT('',#30407);
#8619=VERTEX_POINT('',#30409);
#8620=VERTEX_POINT('',#30411);
#8621=VERTEX_POINT('',#30413);
#8622=VERTEX_POINT('',#30422);
#8623=VERTEX_POINT('',#30423);
#8624=VERTEX_POINT('',#30425);
#8625=VERTEX_POINT('',#30427);
#8626=VERTEX_POINT('',#30431);
#8627=VERTEX_POINT('',#30432);
#8628=VERTEX_POINT('',#30434);
#8629=VERTEX_POINT('',#30436);
#8630=VERTEX_POINT('',#30440);
#8631=VERTEX_POINT('',#30442);
#8632=VERTEX_POINT('',#30444);
#8633=VERTEX_POINT('',#30448);
#8634=VERTEX_POINT('',#30449);
#8635=VERTEX_POINT('',#30451);
#8636=VERTEX_POINT('',#30453);
#8637=VERTEX_POINT('',#30457);
#8638=VERTEX_POINT('',#30458);
#8639=VERTEX_POINT('',#30461);
#8640=VERTEX_POINT('',#30465);
#8641=VERTEX_POINT('',#30466);
#8642=VERTEX_POINT('',#30468);
#8643=VERTEX_POINT('',#30470);
#8644=VERTEX_POINT('',#30477);
#8645=VERTEX_POINT('',#30480);
#8646=VERTEX_POINT('',#30484);
#8647=VERTEX_POINT('',#30489);
#8648=VERTEX_POINT('',#30491);
#8649=VERTEX_POINT('',#30493);
#8650=VERTEX_POINT('',#30497);
#8651=VERTEX_POINT('',#30499);
#8652=VERTEX_POINT('',#30503);
#8653=VERTEX_POINT('',#30505);
#8654=VERTEX_POINT('',#30507);
#8655=VERTEX_POINT('',#30513);
#8656=VERTEX_POINT('',#30514);
#8657=VERTEX_POINT('',#30516);
#8658=VERTEX_POINT('',#30526);
#8659=VERTEX_POINT('',#30527);
#8660=VERTEX_POINT('',#30529);
#8661=VERTEX_POINT('',#30539);
#8662=VERTEX_POINT('',#30540);
#8663=VERTEX_POINT('',#30542);
#8664=VERTEX_POINT('',#30548);
#8665=VERTEX_POINT('',#30550);
#8666=VERTEX_POINT('',#30554);
#8667=VERTEX_POINT('',#30556);
#8668=VERTEX_POINT('',#30560);
#8669=VERTEX_POINT('',#30565);
#8670=VERTEX_POINT('',#30567);
#8671=VERTEX_POINT('',#30572);
#8672=VERTEX_POINT('',#30574);
#8673=VERTEX_POINT('',#30577);
#8674=VERTEX_POINT('',#30580);
#8675=VERTEX_POINT('',#30583);
#8676=VERTEX_POINT('',#30587);
#8677=VERTEX_POINT('',#30591);
#8678=VERTEX_POINT('',#30592);
#8679=VERTEX_POINT('',#30597);
#8680=VERTEX_POINT('',#30601);
#8681=VERTEX_POINT('',#30605);
#8682=VERTEX_POINT('',#30606);
#8683=VERTEX_POINT('',#30608);
#8684=VERTEX_POINT('',#30610);
#8685=VERTEX_POINT('',#30614);
#8686=VERTEX_POINT('',#30619);
#8687=VERTEX_POINT('',#30621);
#8688=VERTEX_POINT('',#30623);
#8689=VERTEX_POINT('',#30625);
#8690=VERTEX_POINT('',#30627);
#8691=VERTEX_POINT('',#30629);
#8692=VERTEX_POINT('',#30631);
#8693=VERTEX_POINT('',#30633);
#8694=VERTEX_POINT('',#30636);
#8695=VERTEX_POINT('',#30638);
#8696=VERTEX_POINT('',#30640);
#8697=VERTEX_POINT('',#30642);
#8698=VERTEX_POINT('',#30645);
#8699=VERTEX_POINT('',#30647);
#8700=VERTEX_POINT('',#30651);
#8701=VERTEX_POINT('',#30653);
#8702=VERTEX_POINT('',#30655);
#8703=VERTEX_POINT('',#30657);
#8704=VERTEX_POINT('',#30659);
#8705=VERTEX_POINT('',#30669);
#8706=VERTEX_POINT('',#30673);
#8707=VERTEX_POINT('',#30679);
#8708=VERTEX_POINT('',#30681);
#8709=VERTEX_POINT('',#30685);
#8710=VERTEX_POINT('',#30686);
#8711=VERTEX_POINT('',#30688);
#8712=VERTEX_POINT('',#30690);
#8713=VERTEX_POINT('',#30694);
#8714=VERTEX_POINT('',#30696);
#8715=VERTEX_POINT('',#30700);
#8716=VERTEX_POINT('',#30702);
#8717=VERTEX_POINT('',#30706);
#8718=VERTEX_POINT('',#30708);
#8719=VERTEX_POINT('',#30712);
#8720=VERTEX_POINT('',#30714);
#8721=VERTEX_POINT('',#30718);
#8722=VERTEX_POINT('',#30720);
#8723=VERTEX_POINT('',#30724);
#8724=VERTEX_POINT('',#30726);
#8725=VERTEX_POINT('',#30737);
#8726=VERTEX_POINT('',#30746);
#8727=VERTEX_POINT('',#30747);
#8728=VERTEX_POINT('',#30749);
#8729=VERTEX_POINT('',#30751);
#8730=VERTEX_POINT('',#30761);
#8731=VERTEX_POINT('',#30762);
#8732=VERTEX_POINT('',#30764);
#8733=VERTEX_POINT('',#30766);
#8734=VERTEX_POINT('',#30773);
#8735=VERTEX_POINT('',#30777);
#8736=VERTEX_POINT('',#30780);
#8737=VERTEX_POINT('',#30784);
#8738=VERTEX_POINT('',#30785);
#8739=VERTEX_POINT('',#30787);
#8740=VERTEX_POINT('',#30789);
#8741=VERTEX_POINT('',#30795);
#8742=VERTEX_POINT('',#30798);
#8743=VERTEX_POINT('',#30803);
#8744=VERTEX_POINT('',#30805);
#8745=VERTEX_POINT('',#30809);
#8746=VERTEX_POINT('',#30812);
#8747=VERTEX_POINT('',#30816);
#8748=VERTEX_POINT('',#30817);
#8749=VERTEX_POINT('',#30822);
#8750=VERTEX_POINT('',#30826);
#8751=VERTEX_POINT('',#30831);
#8752=VERTEX_POINT('',#30836);
#8753=VERTEX_POINT('',#30841);
#8754=VERTEX_POINT('',#30850);
#8755=VERTEX_POINT('',#30852);
#10726=EDGE_CURVE('',#8581,#8582,#1478,.T.);
#10727=EDGE_CURVE('',#8583,#8581,#1479,.T.);
#10728=EDGE_CURVE('',#8584,#8583,#1480,.T.);
#10729=EDGE_CURVE('',#8584,#8582,#1481,.T.);
#10730=EDGE_CURVE('',#8582,#8585,#300,.T.);
#10731=EDGE_CURVE('',#8586,#8584,#7283,.T.);
#10732=EDGE_CURVE('',#8586,#8587,#1482,.T.);
#10733=EDGE_CURVE('',#8585,#8587,#301,.T.);
#10734=EDGE_CURVE('',#8587,#8588,#302,.T.);
#10735=EDGE_CURVE('',#8589,#8586,#7284,.T.);
#10736=EDGE_CURVE('',#8589,#8590,#1483,.T.);
#10737=EDGE_CURVE('',#8591,#8590,#303,.T.);
#10738=EDGE_CURVE('',#8592,#8591,#7285,.T.);
#10739=EDGE_CURVE('',#8593,#8592,#216,.T.);
#10740=EDGE_CURVE('',#8588,#8593,#7286,.T.);
#10741=EDGE_CURVE('',#8590,#8594,#304,.T.);
#10742=EDGE_CURVE('',#8595,#8589,#7287,.T.);
#10743=EDGE_CURVE('',#8595,#8596,#1484,.T.);
#10744=EDGE_CURVE('',#8594,#8596,#305,.T.);
#10745=EDGE_CURVE('',#8596,#8597,#1485,.T.);
#10746=EDGE_CURVE('',#8598,#8595,#1486,.T.);
#10747=EDGE_CURVE('',#8598,#8597,#1487,.T.);
#10748=EDGE_CURVE('',#8597,#8599,#306,.T.);
#10749=EDGE_CURVE('',#8600,#8598,#7288,.T.);
#10750=EDGE_CURVE('',#8600,#8601,#1488,.T.);
#10751=EDGE_CURVE('',#8599,#8601,#307,.T.);
#10752=EDGE_CURVE('',#8601,#8602,#308,.T.);
#10753=EDGE_CURVE('',#8603,#8600,#7289,.T.);
#10754=EDGE_CURVE('',#8603,#8604,#1489,.T.);
#10755=EDGE_CURVE('',#8605,#8604,#309,.T.);
#10756=EDGE_CURVE('',#8606,#8605,#7290,.T.);
#10757=EDGE_CURVE('',#8607,#8606,#217,.T.);
#10758=EDGE_CURVE('',#8602,#8607,#7291,.T.);
#10759=EDGE_CURVE('',#8604,#8608,#310,.T.);
#10760=EDGE_CURVE('',#8609,#8603,#7292,.T.);
#10761=EDGE_CURVE('',#8609,#8610,#1490,.T.);
#10762=EDGE_CURVE('',#8608,#8610,#311,.T.);
#10763=EDGE_CURVE('',#8610,#8611,#1491,.T.);
#10764=EDGE_CURVE('',#8612,#8609,#1492,.T.);
#10765=EDGE_CURVE('',#8612,#8611,#1493,.T.);
#10766=EDGE_CURVE('',#8611,#8613,#312,.T.);
#10767=EDGE_CURVE('',#8614,#8612,#7293,.T.);
#10768=EDGE_CURVE('',#8614,#8615,#1494,.T.);
#10769=EDGE_CURVE('',#8613,#8615,#313,.T.);
#10770=EDGE_CURVE('',#8615,#8616,#314,.T.);
#10771=EDGE_CURVE('',#8617,#8614,#7294,.T.);
#10772=EDGE_CURVE('',#8617,#8618,#1495,.T.);
#10773=EDGE_CURVE('',#8619,#8618,#315,.T.);
#10774=EDGE_CURVE('',#8620,#8619,#7295,.T.);
#10775=EDGE_CURVE('',#8621,#8620,#218,.T.);
#10776=EDGE_CURVE('',#8616,#8621,#7296,.T.);
#10777=EDGE_CURVE('',#8622,#8623,#1496,.T.);
#10778=EDGE_CURVE('',#8622,#8624,#1497,.T.);
#10779=EDGE_CURVE('',#8625,#8624,#1498,.T.);
#10780=EDGE_CURVE('',#8623,#8625,#1499,.T.);
#10781=EDGE_CURVE('',#8626,#8627,#1500,.T.);
#10782=EDGE_CURVE('',#8628,#8626,#1501,.T.);
#10783=EDGE_CURVE('',#8629,#8628,#1502,.T.);
#10784=EDGE_CURVE('',#8629,#8627,#1503,.T.);
#10785=EDGE_CURVE('',#8627,#8630,#1504,.T.);
#10786=EDGE_CURVE('',#8631,#8629,#1505,.T.);
#10787=EDGE_CURVE('',#8632,#8631,#1506,.T.);
#10788=EDGE_CURVE('',#8630,#8632,#1507,.T.);
#10789=EDGE_CURVE('',#8633,#8634,#1508,.T.);
#10790=EDGE_CURVE('',#8635,#8633,#1509,.T.);
#10791=EDGE_CURVE('',#8636,#8635,#1510,.T.);
#10792=EDGE_CURVE('',#8636,#8634,#1511,.T.);
#10793=EDGE_CURVE('',#8637,#8638,#316,.T.);
#10794=EDGE_CURVE('',#8634,#8637,#317,.T.);
#10795=EDGE_CURVE('',#8639,#8636,#7297,.T.);
#10796=EDGE_CURVE('',#8639,#8638,#1512,.T.);
#10797=EDGE_CURVE('',#8640,#8641,#318,.T.);
#10798=EDGE_CURVE('',#8642,#8640,#7298,.T.);
#10799=EDGE_CURVE('',#8643,#8642,#219,.T.);
#10800=EDGE_CURVE('',#8644,#8643,#7299,.T.);
#10801=EDGE_CURVE('',#8638,#8644,#319,.T.);
#10802=EDGE_CURVE('',#8645,#8639,#7300,.T.);
#10803=EDGE_CURVE('',#8645,#8641,#1513,.T.);
#10804=EDGE_CURVE('',#8646,#8581,#320,.T.);
#10805=EDGE_CURVE('',#8641,#8646,#321,.T.);
#10806=EDGE_CURVE('',#8583,#8645,#7301,.T.);
#10807=EDGE_CURVE('',#8647,#8617,#7302,.T.);
#10808=EDGE_CURVE('',#8647,#8648,#1514,.T.);
#10809=EDGE_CURVE('',#8649,#8648,#322,.T.);
#10810=EDGE_CURVE('',#8618,#8649,#323,.T.);
#10811=EDGE_CURVE('',#8650,#8647,#1515,.T.);
#10812=EDGE_CURVE('',#8651,#8650,#1516,.T.);
#10813=EDGE_CURVE('',#8648,#8651,#1517,.T.);
#10814=EDGE_CURVE('',#8652,#8622,#1518,.T.);
#10815=EDGE_CURVE('',#8653,#8652,#1519,.T.);
#10816=EDGE_CURVE('',#8654,#8653,#1520,.T.);
#10817=EDGE_CURVE('',#8624,#8654,#1521,.T.);
#10818=EDGE_CURVE('',#8646,#8585,#1522,.T.);
#10819=EDGE_CURVE('',#8655,#8656,#7303,.T.);
#10820=EDGE_CURVE('',#8656,#8657,#1523,.T.);
#10821=EDGE_CURVE('',#8657,#8593,#7304,.T.);
#10822=EDGE_CURVE('',#8592,#8657,#7305,.T.);
#10823=EDGE_CURVE('',#8656,#8655,#7306,.T.);
#10824=EDGE_CURVE('',#8594,#8599,#1524,.T.);
#10825=EDGE_CURVE('',#8602,#8591,#1525,.T.);
#10826=EDGE_CURVE('',#8658,#8659,#7307,.T.);
#10827=EDGE_CURVE('',#8659,#8660,#1526,.T.);
#10828=EDGE_CURVE('',#8660,#8607,#7308,.T.);
#10829=EDGE_CURVE('',#8606,#8660,#7309,.T.);
#10830=EDGE_CURVE('',#8659,#8658,#7310,.T.);
#10831=EDGE_CURVE('',#8608,#8613,#1527,.T.);
#10832=EDGE_CURVE('',#8616,#8605,#1528,.T.);
#10833=EDGE_CURVE('',#8661,#8662,#7311,.T.);
#10834=EDGE_CURVE('',#8662,#8663,#1529,.T.);
#10835=EDGE_CURVE('',#8663,#8621,#7312,.T.);
#10836=EDGE_CURVE('',#8620,#8663,#7313,.T.);
#10837=EDGE_CURVE('',#8662,#8661,#7314,.T.);
#10838=EDGE_CURVE('',#8664,#8649,#1530,.T.);
#10839=EDGE_CURVE('',#8665,#8664,#1531,.T.);
#10840=EDGE_CURVE('',#8665,#8619,#1532,.T.);
#10841=EDGE_CURVE('',#8666,#8625,#1533,.T.);
#10842=EDGE_CURVE('',#8667,#8666,#1534,.T.);
#10843=EDGE_CURVE('',#8667,#8623,#1535,.T.);
#10844=EDGE_CURVE('',#8654,#8668,#1536,.T.);
#10845=EDGE_CURVE('',#8668,#8665,#1537,.T.);
#10846=EDGE_CURVE('',#8664,#8666,#1538,.T.);
#10847=EDGE_CURVE('',#8632,#8669,#1539,.T.);
#10848=EDGE_CURVE('',#8669,#8670,#1540,.T.);
#10849=EDGE_CURVE('',#8670,#8630,#1541,.T.);
#10850=EDGE_CURVE('',#8588,#8640,#1542,.T.);
#10851=EDGE_CURVE('',#8671,#8668,#1543,.T.);
#10852=EDGE_CURVE('',#8672,#8671,#1544,.T.);
#10853=EDGE_CURVE('',#8644,#8672,#1545,.T.);
#10854=EDGE_CURVE('',#8673,#8643,#7315,.T.);
#10855=EDGE_CURVE('',#8642,#8673,#7316,.T.);
#10856=EDGE_CURVE('',#8674,#8674,#7317,.T.);
#10857=EDGE_CURVE('',#8675,#8675,#7318,.T.);
#10858=EDGE_CURVE('',#8675,#8658,#1546,.T.);
#10859=EDGE_CURVE('',#8676,#8676,#7319,.T.);
#10860=EDGE_CURVE('',#8676,#8661,#1547,.T.);
#10861=EDGE_CURVE('',#8677,#8678,#7320,.T.);
#10862=EDGE_CURVE('',#8678,#8673,#1548,.T.);
#10863=EDGE_CURVE('',#8678,#8677,#7321,.T.);
#10864=EDGE_CURVE('',#8679,#8679,#7322,.T.);
#10865=EDGE_CURVE('',#8679,#8677,#1549,.T.);
#10866=EDGE_CURVE('',#8680,#8680,#7323,.T.);
#10867=EDGE_CURVE('',#8680,#8655,#1550,.T.);
#10868=EDGE_CURVE('',#8681,#8682,#7324,.T.);
#10869=EDGE_CURVE('',#8682,#8683,#1551,.T.);
#10870=EDGE_CURVE('',#8683,#8684,#7325,.T.);
#10871=EDGE_CURVE('',#8684,#8681,#1552,.T.);
#10872=EDGE_CURVE('',#8685,#8633,#1553,.T.);
#10873=EDGE_CURVE('',#8685,#8683,#1554,.T.);
#10874=EDGE_CURVE('',#8635,#8682,#1555,.T.);
#10875=EDGE_CURVE('',#8681,#8686,#1556,.T.);
#10876=EDGE_CURVE('',#8686,#8687,#1557,.T.);
#10877=EDGE_CURVE('',#8687,#8688,#1558,.T.);
#10878=EDGE_CURVE('',#8688,#8689,#1559,.T.);
#10879=EDGE_CURVE('',#8689,#8690,#1560,.T.);
#10880=EDGE_CURVE('',#8690,#8691,#1561,.T.);
#10881=EDGE_CURVE('',#8691,#8692,#1562,.T.);
#10882=EDGE_CURVE('',#8693,#8692,#7326,.T.);
#10883=EDGE_CURVE('',#8693,#8650,#1563,.T.);
#10884=EDGE_CURVE('',#8694,#8694,#7327,.T.);
#10885=EDGE_CURVE('',#8695,#8695,#7328,.T.);
#10886=EDGE_CURVE('',#8696,#8696,#7329,.T.);
#10887=EDGE_CURVE('',#8697,#8697,#7330,.T.);
#10888=EDGE_CURVE('',#8692,#8698,#1564,.T.);
#10889=EDGE_CURVE('',#8698,#8699,#7331,.T.);
#10890=EDGE_CURVE('',#8699,#8693,#1565,.T.);
#10891=EDGE_CURVE('',#8691,#8700,#1566,.T.);
#10892=EDGE_CURVE('',#8700,#8701,#1567,.T.);
#10893=EDGE_CURVE('',#8701,#8702,#1568,.T.);
#10894=EDGE_CURVE('',#8702,#8703,#1569,.T.);
#10895=EDGE_CURVE('',#8703,#8704,#1570,.T.);
#10896=EDGE_CURVE('',#8704,#8698,#1571,.T.);
#10897=EDGE_CURVE('',#8699,#8667,#1572,.T.);
#10898=EDGE_CURVE('',#8651,#8667,#1573,.T.);
#10899=EDGE_CURVE('',#8671,#8631,#1574,.T.);
#10900=EDGE_CURVE('',#8669,#8671,#1575,.T.);
#10901=EDGE_CURVE('',#8705,#8653,#1576,.T.);
#10902=EDGE_CURVE('',#8668,#8705,#1577,.T.);
#10903=EDGE_CURVE('',#8652,#8706,#1578,.T.);
#10904=EDGE_CURVE('',#8706,#8705,#1579,.T.);
#10905=EDGE_CURVE('',#8705,#8669,#1580,.T.);
#10906=EDGE_CURVE('',#8628,#8707,#1581,.T.);
#10907=EDGE_CURVE('',#8708,#8707,#1582,.T.);
#10908=EDGE_CURVE('',#8672,#8708,#1583,.T.);
#10909=EDGE_CURVE('',#8709,#8710,#7332,.T.);
#10910=EDGE_CURVE('',#8709,#8711,#1584,.T.);
#10911=EDGE_CURVE('',#8711,#8712,#7333,.T.);
#10912=EDGE_CURVE('',#8712,#8710,#1585,.T.);
#10913=EDGE_CURVE('',#8709,#8713,#1586,.T.);
#10914=EDGE_CURVE('',#8714,#8713,#1587,.T.);
#10915=EDGE_CURVE('',#8711,#8714,#1588,.T.);
#10916=EDGE_CURVE('',#8715,#8713,#7334,.T.);
#10917=EDGE_CURVE('',#8715,#8716,#1589,.T.);
#10918=EDGE_CURVE('',#8716,#8714,#7335,.T.);
#10919=EDGE_CURVE('',#8715,#8717,#1590,.T.);
#10920=EDGE_CURVE('',#8718,#8717,#1591,.T.);
#10921=EDGE_CURVE('',#8716,#8718,#1592,.T.);
#10922=EDGE_CURVE('',#8719,#8717,#7336,.T.);
#10923=EDGE_CURVE('',#8719,#8720,#1593,.T.);
#10924=EDGE_CURVE('',#8720,#8718,#7337,.T.);
#10925=EDGE_CURVE('',#8719,#8721,#1594,.T.);
#10926=EDGE_CURVE('',#8722,#8721,#1595,.T.);
#10927=EDGE_CURVE('',#8720,#8722,#1596,.T.);
#10928=EDGE_CURVE('',#8723,#8721,#7338,.T.);
#10929=EDGE_CURVE('',#8723,#8724,#1597,.T.);
#10930=EDGE_CURVE('',#8724,#8722,#7339,.T.);
#10931=EDGE_CURVE('',#8723,#8710,#1598,.T.);
#10932=EDGE_CURVE('',#8724,#8712,#1599,.T.);
#10933=EDGE_CURVE('',#8708,#8637,#1600,.T.);
#10934=EDGE_CURVE('',#8725,#8725,#7340,.T.);
#10935=EDGE_CURVE('',#8725,#8674,#1601,.T.);
#10936=EDGE_CURVE('',#8626,#8685,#1602,.T.);
#10937=EDGE_CURVE('',#8707,#8685,#1603,.T.);
#10938=EDGE_CURVE('',#8706,#8670,#1604,.T.);
#10939=EDGE_CURVE('',#8726,#8727,#7341,.T.);
#10940=EDGE_CURVE('',#8728,#8726,#1605,.T.);
#10941=EDGE_CURVE('',#8729,#8728,#7342,.T.);
#10942=EDGE_CURVE('',#8727,#8729,#1606,.T.);
#10943=EDGE_CURVE('',#8729,#8728,#1607,.T.);
#10944=EDGE_CURVE('',#8704,#8701,#7343,.T.);
#10945=EDGE_CURVE('',#8702,#8703,#7344,.T.);
#10946=EDGE_CURVE('',#8730,#8731,#7345,.T.);
#10947=EDGE_CURVE('',#8732,#8730,#1608,.T.);
#10948=EDGE_CURVE('',#8733,#8732,#7346,.T.);
#10949=EDGE_CURVE('',#8731,#8733,#1609,.T.);
#10950=EDGE_CURVE('',#8733,#8732,#1610,.T.);
#10951=EDGE_CURVE('',#8684,#8727,#1611,.T.);
#10952=EDGE_CURVE('',#8726,#8734,#1612,.T.);
#10953=EDGE_CURVE('',#8686,#8734,#1613,.T.);
#10954=EDGE_CURVE('',#8730,#8735,#1614,.T.);
#10955=EDGE_CURVE('',#8690,#8735,#1615,.T.);
#10956=EDGE_CURVE('',#8689,#8736,#1616,.T.);
#10957=EDGE_CURVE('',#8736,#8731,#1617,.T.);
#10958=EDGE_CURVE('',#8737,#8738,#7347,.T.);
#10959=EDGE_CURVE('',#8739,#8737,#1618,.T.);
#10960=EDGE_CURVE('',#8740,#8739,#7348,.T.);
#10961=EDGE_CURVE('',#8738,#8740,#1619,.T.);
#10962=EDGE_CURVE('',#8740,#8739,#1620,.T.);
#10963=EDGE_CURVE('',#8737,#8741,#1621,.T.);
#10964=EDGE_CURVE('',#8688,#8741,#1622,.T.);
#10965=EDGE_CURVE('',#8687,#8742,#1623,.T.);
#10966=EDGE_CURVE('',#8742,#8738,#1624,.T.);
#10967=EDGE_CURVE('',#8743,#8743,#7349,.T.);
#10968=EDGE_CURVE('',#8743,#8744,#1625,.T.);
#10969=EDGE_CURVE('',#8744,#8744,#7350,.T.);
#10970=EDGE_CURVE('',#8745,#8745,#7351,.T.);
#10971=EDGE_CURVE('',#8746,#8746,#7352,.T.);
#10972=EDGE_CURVE('',#8746,#8743,#1626,.T.);
#10973=EDGE_CURVE('',#8747,#8748,#7353,.T.);
#10974=EDGE_CURVE('',#8748,#8745,#1627,.T.);
#10975=EDGE_CURVE('',#8748,#8747,#7354,.T.);
#10976=EDGE_CURVE('',#8747,#8749,#1628,.T.);
#10977=EDGE_CURVE('',#8749,#8749,#7355,.T.);
#10978=EDGE_CURVE('',#8750,#8750,#7356,.T.);
#10979=EDGE_CURVE('',#8694,#8750,#1629,.T.);
#10980=EDGE_CURVE('',#8751,#8751,#7357,.T.);
#10981=EDGE_CURVE('',#8695,#8751,#1630,.T.);
#10982=EDGE_CURVE('',#8752,#8752,#7358,.T.);
#10983=EDGE_CURVE('',#8696,#8752,#1631,.T.);
#10984=EDGE_CURVE('',#8753,#8753,#7359,.T.);
#10985=EDGE_CURVE('',#8697,#8753,#1632,.T.);
#10986=EDGE_CURVE('',#8735,#8700,#1633,.T.);
#10987=EDGE_CURVE('',#8741,#8736,#1634,.T.);
#10988=EDGE_CURVE('',#8734,#8742,#1635,.T.);
#10989=EDGE_CURVE('',#8754,#8754,#7360,.T.);
#10990=EDGE_CURVE('',#8754,#8755,#1636,.T.);
#10991=EDGE_CURVE('',#8755,#8755,#7361,.T.);
#14336=ORIENTED_EDGE('',*,*,#10726,.F.);
#14337=ORIENTED_EDGE('',*,*,#10727,.F.);
#14338=ORIENTED_EDGE('',*,*,#10728,.F.);
#14339=ORIENTED_EDGE('',*,*,#10729,.T.);
#14340=ORIENTED_EDGE('',*,*,#10730,.F.);
#14341=ORIENTED_EDGE('',*,*,#10729,.F.);
#14342=ORIENTED_EDGE('',*,*,#10731,.F.);
#14343=ORIENTED_EDGE('',*,*,#10732,.T.);
#14344=ORIENTED_EDGE('',*,*,#10733,.F.);
#14345=ORIENTED_EDGE('',*,*,#10734,.F.);
#14346=ORIENTED_EDGE('',*,*,#10732,.F.);
#14347=ORIENTED_EDGE('',*,*,#10735,.F.);
#14348=ORIENTED_EDGE('',*,*,#10736,.T.);
#14349=ORIENTED_EDGE('',*,*,#10737,.F.);
#14350=ORIENTED_EDGE('',*,*,#10738,.F.);
#14351=ORIENTED_EDGE('',*,*,#10739,.F.);
#14352=ORIENTED_EDGE('',*,*,#10740,.F.);
#14353=ORIENTED_EDGE('',*,*,#10741,.F.);
#14354=ORIENTED_EDGE('',*,*,#10736,.F.);
#14355=ORIENTED_EDGE('',*,*,#10742,.F.);
#14356=ORIENTED_EDGE('',*,*,#10743,.T.);
#14357=ORIENTED_EDGE('',*,*,#10744,.F.);
#14358=ORIENTED_EDGE('',*,*,#10745,.F.);
#14359=ORIENTED_EDGE('',*,*,#10743,.F.);
#14360=ORIENTED_EDGE('',*,*,#10746,.F.);
#14361=ORIENTED_EDGE('',*,*,#10747,.T.);
#14362=ORIENTED_EDGE('',*,*,#10748,.F.);
#14363=ORIENTED_EDGE('',*,*,#10747,.F.);
#14364=ORIENTED_EDGE('',*,*,#10749,.F.);
#14365=ORIENTED_EDGE('',*,*,#10750,.T.);
#14366=ORIENTED_EDGE('',*,*,#10751,.F.);
#14367=ORIENTED_EDGE('',*,*,#10752,.F.);
#14368=ORIENTED_EDGE('',*,*,#10750,.F.);
#14369=ORIENTED_EDGE('',*,*,#10753,.F.);
#14370=ORIENTED_EDGE('',*,*,#10754,.T.);
#14371=ORIENTED_EDGE('',*,*,#10755,.F.);
#14372=ORIENTED_EDGE('',*,*,#10756,.F.);
#14373=ORIENTED_EDGE('',*,*,#10757,.F.);
#14374=ORIENTED_EDGE('',*,*,#10758,.F.);
#14375=ORIENTED_EDGE('',*,*,#10759,.F.);
#14376=ORIENTED_EDGE('',*,*,#10754,.F.);
#14377=ORIENTED_EDGE('',*,*,#10760,.F.);
#14378=ORIENTED_EDGE('',*,*,#10761,.T.);
#14379=ORIENTED_EDGE('',*,*,#10762,.F.);
#14380=ORIENTED_EDGE('',*,*,#10763,.F.);
#14381=ORIENTED_EDGE('',*,*,#10761,.F.);
#14382=ORIENTED_EDGE('',*,*,#10764,.F.);
#14383=ORIENTED_EDGE('',*,*,#10765,.T.);
#14384=ORIENTED_EDGE('',*,*,#10766,.F.);
#14385=ORIENTED_EDGE('',*,*,#10765,.F.);
#14386=ORIENTED_EDGE('',*,*,#10767,.F.);
#14387=ORIENTED_EDGE('',*,*,#10768,.T.);
#14388=ORIENTED_EDGE('',*,*,#10769,.F.);
#14389=ORIENTED_EDGE('',*,*,#10770,.F.);
#14390=ORIENTED_EDGE('',*,*,#10768,.F.);
#14391=ORIENTED_EDGE('',*,*,#10771,.F.);
#14392=ORIENTED_EDGE('',*,*,#10772,.T.);
#14393=ORIENTED_EDGE('',*,*,#10773,.F.);
#14394=ORIENTED_EDGE('',*,*,#10774,.F.);
#14395=ORIENTED_EDGE('',*,*,#10775,.F.);
#14396=ORIENTED_EDGE('',*,*,#10776,.F.);
#14397=ORIENTED_EDGE('',*,*,#10777,.F.);
#14398=ORIENTED_EDGE('',*,*,#10778,.T.);
#14399=ORIENTED_EDGE('',*,*,#10779,.F.);
#14400=ORIENTED_EDGE('',*,*,#10780,.F.);
#14401=ORIENTED_EDGE('',*,*,#10781,.F.);
#14402=ORIENTED_EDGE('',*,*,#10782,.F.);
#14403=ORIENTED_EDGE('',*,*,#10783,.F.);
#14404=ORIENTED_EDGE('',*,*,#10784,.T.);
#14405=ORIENTED_EDGE('',*,*,#10785,.F.);
#14406=ORIENTED_EDGE('',*,*,#10784,.F.);
#14407=ORIENTED_EDGE('',*,*,#10786,.F.);
#14408=ORIENTED_EDGE('',*,*,#10787,.F.);
#14409=ORIENTED_EDGE('',*,*,#10788,.F.);
#14410=ORIENTED_EDGE('',*,*,#10789,.F.);
#14411=ORIENTED_EDGE('',*,*,#10790,.F.);
#14412=ORIENTED_EDGE('',*,*,#10791,.F.);
#14413=ORIENTED_EDGE('',*,*,#10792,.T.);
#14414=ORIENTED_EDGE('',*,*,#10793,.F.);
#14415=ORIENTED_EDGE('',*,*,#10794,.F.);
#14416=ORIENTED_EDGE('',*,*,#10792,.F.);
#14417=ORIENTED_EDGE('',*,*,#10795,.F.);
#14418=ORIENTED_EDGE('',*,*,#10796,.T.);
#14419=ORIENTED_EDGE('',*,*,#10797,.F.);
#14420=ORIENTED_EDGE('',*,*,#10798,.F.);
#14421=ORIENTED_EDGE('',*,*,#10799,.F.);
#14422=ORIENTED_EDGE('',*,*,#10800,.F.);
#14423=ORIENTED_EDGE('',*,*,#10801,.F.);
#14424=ORIENTED_EDGE('',*,*,#10796,.F.);
#14425=ORIENTED_EDGE('',*,*,#10802,.F.);
#14426=ORIENTED_EDGE('',*,*,#10803,.T.);
#14427=ORIENTED_EDGE('',*,*,#10804,.F.);
#14428=ORIENTED_EDGE('',*,*,#10805,.F.);
#14429=ORIENTED_EDGE('',*,*,#10803,.F.);
#14430=ORIENTED_EDGE('',*,*,#10806,.F.);
#14431=ORIENTED_EDGE('',*,*,#10727,.T.);
#14432=ORIENTED_EDGE('',*,*,#10807,.F.);
#14433=ORIENTED_EDGE('',*,*,#10808,.T.);
#14434=ORIENTED_EDGE('',*,*,#10809,.F.);
#14435=ORIENTED_EDGE('',*,*,#10810,.F.);
#14436=ORIENTED_EDGE('',*,*,#10772,.F.);
#14437=ORIENTED_EDGE('',*,*,#10811,.F.);
#14438=ORIENTED_EDGE('',*,*,#10812,.F.);
#14439=ORIENTED_EDGE('',*,*,#10813,.F.);
#14440=ORIENTED_EDGE('',*,*,#10808,.F.);
#14441=ORIENTED_EDGE('',*,*,#10814,.F.);
#14442=ORIENTED_EDGE('',*,*,#10815,.F.);
#14443=ORIENTED_EDGE('',*,*,#10816,.F.);
#14444=ORIENTED_EDGE('',*,*,#10817,.F.);
#14445=ORIENTED_EDGE('',*,*,#10778,.F.);
#14446=ORIENTED_EDGE('',*,*,#10804,.T.);
#14447=ORIENTED_EDGE('',*,*,#10726,.T.);
#14448=ORIENTED_EDGE('',*,*,#10730,.T.);
#14449=ORIENTED_EDGE('',*,*,#10818,.F.);
#14450=ORIENTED_EDGE('',*,*,#10819,.T.);
#14451=ORIENTED_EDGE('',*,*,#10820,.T.);
#14452=ORIENTED_EDGE('',*,*,#10821,.T.);
#14453=ORIENTED_EDGE('',*,*,#10739,.T.);
#14454=ORIENTED_EDGE('',*,*,#10822,.T.);
#14455=ORIENTED_EDGE('',*,*,#10820,.F.);
#14456=ORIENTED_EDGE('',*,*,#10823,.T.);
#14457=ORIENTED_EDGE('',*,*,#10744,.T.);
#14458=ORIENTED_EDGE('',*,*,#10745,.T.);
#14459=ORIENTED_EDGE('',*,*,#10748,.T.);
#14460=ORIENTED_EDGE('',*,*,#10824,.F.);
#14461=ORIENTED_EDGE('',*,*,#10737,.T.);
#14462=ORIENTED_EDGE('',*,*,#10741,.T.);
#14463=ORIENTED_EDGE('',*,*,#10824,.T.);
#14464=ORIENTED_EDGE('',*,*,#10751,.T.);
#14465=ORIENTED_EDGE('',*,*,#10752,.T.);
#14466=ORIENTED_EDGE('',*,*,#10825,.T.);
#14467=ORIENTED_EDGE('',*,*,#10826,.T.);
#14468=ORIENTED_EDGE('',*,*,#10827,.T.);
#14469=ORIENTED_EDGE('',*,*,#10828,.T.);
#14470=ORIENTED_EDGE('',*,*,#10757,.T.);
#14471=ORIENTED_EDGE('',*,*,#10829,.T.);
#14472=ORIENTED_EDGE('',*,*,#10827,.F.);
#14473=ORIENTED_EDGE('',*,*,#10830,.T.);
#14474=ORIENTED_EDGE('',*,*,#10762,.T.);
#14475=ORIENTED_EDGE('',*,*,#10763,.T.);
#14476=ORIENTED_EDGE('',*,*,#10766,.T.);
#14477=ORIENTED_EDGE('',*,*,#10831,.F.);
#14478=ORIENTED_EDGE('',*,*,#10755,.T.);
#14479=ORIENTED_EDGE('',*,*,#10759,.T.);
#14480=ORIENTED_EDGE('',*,*,#10831,.T.);
#14481=ORIENTED_EDGE('',*,*,#10769,.T.);
#14482=ORIENTED_EDGE('',*,*,#10770,.T.);
#14483=ORIENTED_EDGE('',*,*,#10832,.T.);
#14484=ORIENTED_EDGE('',*,*,#10833,.T.);
#14485=ORIENTED_EDGE('',*,*,#10834,.T.);
#14486=ORIENTED_EDGE('',*,*,#10835,.T.);
#14487=ORIENTED_EDGE('',*,*,#10775,.T.);
#14488=ORIENTED_EDGE('',*,*,#10836,.T.);
#14489=ORIENTED_EDGE('',*,*,#10834,.F.);
#14490=ORIENTED_EDGE('',*,*,#10837,.T.);
#14491=ORIENTED_EDGE('',*,*,#10773,.T.);
#14492=ORIENTED_EDGE('',*,*,#10810,.T.);
#14493=ORIENTED_EDGE('',*,*,#10838,.F.);
#14494=ORIENTED_EDGE('',*,*,#10839,.F.);
#14495=ORIENTED_EDGE('',*,*,#10840,.T.);
#14496=ORIENTED_EDGE('',*,*,#10780,.T.);
#14497=ORIENTED_EDGE('',*,*,#10841,.F.);
#14498=ORIENTED_EDGE('',*,*,#10842,.F.);
#14499=ORIENTED_EDGE('',*,*,#10843,.T.);
#14500=ORIENTED_EDGE('',*,*,#10779,.T.);
#14501=ORIENTED_EDGE('',*,*,#10817,.T.);
#14502=ORIENTED_EDGE('',*,*,#10844,.T.);
#14503=ORIENTED_EDGE('',*,*,#10845,.T.);
#14504=ORIENTED_EDGE('',*,*,#10839,.T.);
#14505=ORIENTED_EDGE('',*,*,#10846,.T.);
#14506=ORIENTED_EDGE('',*,*,#10841,.T.);
#14507=ORIENTED_EDGE('',*,*,#10788,.T.);
#14508=ORIENTED_EDGE('',*,*,#10847,.T.);
#14509=ORIENTED_EDGE('',*,*,#10848,.T.);
#14510=ORIENTED_EDGE('',*,*,#10849,.T.);
#14511=ORIENTED_EDGE('',*,*,#10798,.T.);
#14512=ORIENTED_EDGE('',*,*,#10850,.F.);
#14513=ORIENTED_EDGE('',*,*,#10740,.T.);
#14514=ORIENTED_EDGE('',*,*,#10821,.F.);
#14515=ORIENTED_EDGE('',*,*,#10822,.F.);
#14516=ORIENTED_EDGE('',*,*,#10738,.T.);
#14517=ORIENTED_EDGE('',*,*,#10825,.F.);
#14518=ORIENTED_EDGE('',*,*,#10758,.T.);
#14519=ORIENTED_EDGE('',*,*,#10828,.F.);
#14520=ORIENTED_EDGE('',*,*,#10829,.F.);
#14521=ORIENTED_EDGE('',*,*,#10756,.T.);
#14522=ORIENTED_EDGE('',*,*,#10832,.F.);
#14523=ORIENTED_EDGE('',*,*,#10776,.T.);
#14524=ORIENTED_EDGE('',*,*,#10835,.F.);
#14525=ORIENTED_EDGE('',*,*,#10836,.F.);
#14526=ORIENTED_EDGE('',*,*,#10774,.T.);
#14527=ORIENTED_EDGE('',*,*,#10840,.F.);
#14528=ORIENTED_EDGE('',*,*,#10845,.F.);
#14529=ORIENTED_EDGE('',*,*,#10851,.F.);
#14530=ORIENTED_EDGE('',*,*,#10852,.F.);
#14531=ORIENTED_EDGE('',*,*,#10853,.F.);
#14532=ORIENTED_EDGE('',*,*,#10800,.T.);
#14533=ORIENTED_EDGE('',*,*,#10854,.F.);
#14534=ORIENTED_EDGE('',*,*,#10855,.F.);
#14535=ORIENTED_EDGE('',*,*,#10856,.T.);
#14536=ORIENTED_EDGE('',*,*,#10857,.F.);
#14537=ORIENTED_EDGE('',*,*,#10858,.T.);
#14538=ORIENTED_EDGE('',*,*,#10830,.F.);
#14539=ORIENTED_EDGE('',*,*,#10826,.F.);
#14540=ORIENTED_EDGE('',*,*,#10858,.F.);
#14541=ORIENTED_EDGE('',*,*,#10859,.F.);
#14542=ORIENTED_EDGE('',*,*,#10860,.T.);
#14543=ORIENTED_EDGE('',*,*,#10837,.F.);
#14544=ORIENTED_EDGE('',*,*,#10833,.F.);
#14545=ORIENTED_EDGE('',*,*,#10860,.F.);
#14546=ORIENTED_EDGE('',*,*,#10861,.T.);
#14547=ORIENTED_EDGE('',*,*,#10862,.T.);
#14548=ORIENTED_EDGE('',*,*,#10854,.T.);
#14549=ORIENTED_EDGE('',*,*,#10799,.T.);
#14550=ORIENTED_EDGE('',*,*,#10855,.T.);
#14551=ORIENTED_EDGE('',*,*,#10862,.F.);
#14552=ORIENTED_EDGE('',*,*,#10863,.T.);
#14553=ORIENTED_EDGE('',*,*,#10864,.F.);
#14554=ORIENTED_EDGE('',*,*,#10865,.T.);
#14555=ORIENTED_EDGE('',*,*,#10863,.F.);
#14556=ORIENTED_EDGE('',*,*,#10861,.F.);
#14557=ORIENTED_EDGE('',*,*,#10865,.F.);
#14558=ORIENTED_EDGE('',*,*,#10866,.F.);
#14559=ORIENTED_EDGE('',*,*,#10867,.T.);
#14560=ORIENTED_EDGE('',*,*,#10823,.F.);
#14561=ORIENTED_EDGE('',*,*,#10819,.F.);
#14562=ORIENTED_EDGE('',*,*,#10867,.F.);
#14563=ORIENTED_EDGE('',*,*,#10868,.T.);
#14564=ORIENTED_EDGE('',*,*,#10869,.T.);
#14565=ORIENTED_EDGE('',*,*,#10870,.T.);
#14566=ORIENTED_EDGE('',*,*,#10871,.T.);
#14567=ORIENTED_EDGE('',*,*,#10790,.T.);
#14568=ORIENTED_EDGE('',*,*,#10872,.F.);
#14569=ORIENTED_EDGE('',*,*,#10873,.T.);
#14570=ORIENTED_EDGE('',*,*,#10869,.F.);
#14571=ORIENTED_EDGE('',*,*,#10874,.F.);
#14572=ORIENTED_EDGE('',*,*,#10791,.T.);
#14573=ORIENTED_EDGE('',*,*,#10874,.T.);
#14574=ORIENTED_EDGE('',*,*,#10868,.F.);
#14575=ORIENTED_EDGE('',*,*,#10875,.T.);
#14576=ORIENTED_EDGE('',*,*,#10876,.T.);
#14577=ORIENTED_EDGE('',*,*,#10877,.T.);
#14578=ORIENTED_EDGE('',*,*,#10878,.T.);
#14579=ORIENTED_EDGE('',*,*,#10879,.T.);
#14580=ORIENTED_EDGE('',*,*,#10880,.T.);
#14581=ORIENTED_EDGE('',*,*,#10881,.T.);
#14582=ORIENTED_EDGE('',*,*,#10882,.F.);
#14583=ORIENTED_EDGE('',*,*,#10883,.T.);
#14584=ORIENTED_EDGE('',*,*,#10811,.T.);
#14585=ORIENTED_EDGE('',*,*,#10807,.T.);
#14586=ORIENTED_EDGE('',*,*,#10771,.T.);
#14587=ORIENTED_EDGE('',*,*,#10767,.T.);
#14588=ORIENTED_EDGE('',*,*,#10764,.T.);
#14589=ORIENTED_EDGE('',*,*,#10760,.T.);
#14590=ORIENTED_EDGE('',*,*,#10753,.T.);
#14591=ORIENTED_EDGE('',*,*,#10749,.T.);
#14592=ORIENTED_EDGE('',*,*,#10746,.T.);
#14593=ORIENTED_EDGE('',*,*,#10742,.T.);
#14594=ORIENTED_EDGE('',*,*,#10735,.T.);
#14595=ORIENTED_EDGE('',*,*,#10731,.T.);
#14596=ORIENTED_EDGE('',*,*,#10728,.T.);
#14597=ORIENTED_EDGE('',*,*,#10806,.T.);
#14598=ORIENTED_EDGE('',*,*,#10802,.T.);
#14599=ORIENTED_EDGE('',*,*,#10795,.T.);
#14600=ORIENTED_EDGE('',*,*,#10884,.T.);
#14601=ORIENTED_EDGE('',*,*,#10885,.T.);
#14602=ORIENTED_EDGE('',*,*,#10886,.T.);
#14603=ORIENTED_EDGE('',*,*,#10887,.T.);
#14604=ORIENTED_EDGE('',*,*,#10882,.T.);
#14605=ORIENTED_EDGE('',*,*,#10888,.T.);
#14606=ORIENTED_EDGE('',*,*,#10889,.T.);
#14607=ORIENTED_EDGE('',*,*,#10890,.T.);
#14608=ORIENTED_EDGE('',*,*,#10888,.F.);
#14609=ORIENTED_EDGE('',*,*,#10881,.F.);
#14610=ORIENTED_EDGE('',*,*,#10891,.T.);
#14611=ORIENTED_EDGE('',*,*,#10892,.T.);
#14612=ORIENTED_EDGE('',*,*,#10893,.T.);
#14613=ORIENTED_EDGE('',*,*,#10894,.T.);
#14614=ORIENTED_EDGE('',*,*,#10895,.T.);
#14615=ORIENTED_EDGE('',*,*,#10896,.T.);
#14616=ORIENTED_EDGE('',*,*,#10812,.T.);
#14617=ORIENTED_EDGE('',*,*,#10883,.F.);
#14618=ORIENTED_EDGE('',*,*,#10890,.F.);
#14619=ORIENTED_EDGE('',*,*,#10897,.T.);
#14620=ORIENTED_EDGE('',*,*,#10898,.F.);
#14621=ORIENTED_EDGE('',*,*,#10787,.T.);
#14622=ORIENTED_EDGE('',*,*,#10899,.F.);
#14623=ORIENTED_EDGE('',*,*,#10900,.F.);
#14624=ORIENTED_EDGE('',*,*,#10847,.F.);
#14625=ORIENTED_EDGE('',*,*,#10816,.T.);
#14626=ORIENTED_EDGE('',*,*,#10901,.F.);
#14627=ORIENTED_EDGE('',*,*,#10902,.F.);
#14628=ORIENTED_EDGE('',*,*,#10844,.F.);
#14629=ORIENTED_EDGE('',*,*,#10815,.T.);
#14630=ORIENTED_EDGE('',*,*,#10903,.T.);
#14631=ORIENTED_EDGE('',*,*,#10904,.T.);
#14632=ORIENTED_EDGE('',*,*,#10901,.T.);
#14633=ORIENTED_EDGE('',*,*,#10900,.T.);
#14634=ORIENTED_EDGE('',*,*,#10851,.T.);
#14635=ORIENTED_EDGE('',*,*,#10902,.T.);
#14636=ORIENTED_EDGE('',*,*,#10905,.T.);
#14637=ORIENTED_EDGE('',*,*,#10783,.T.);
#14638=ORIENTED_EDGE('',*,*,#10906,.T.);
#14639=ORIENTED_EDGE('',*,*,#10907,.F.);
#14640=ORIENTED_EDGE('',*,*,#10908,.F.);
#14641=ORIENTED_EDGE('',*,*,#10852,.T.);
#14642=ORIENTED_EDGE('',*,*,#10899,.T.);
#14643=ORIENTED_EDGE('',*,*,#10786,.T.);
#14644=ORIENTED_EDGE('',*,*,#10909,.F.);
#14645=ORIENTED_EDGE('',*,*,#10910,.T.);
#14646=ORIENTED_EDGE('',*,*,#10911,.T.);
#14647=ORIENTED_EDGE('',*,*,#10912,.T.);
#14648=ORIENTED_EDGE('',*,*,#10910,.F.);
#14649=ORIENTED_EDGE('',*,*,#10913,.T.);
#14650=ORIENTED_EDGE('',*,*,#10914,.F.);
#14651=ORIENTED_EDGE('',*,*,#10915,.F.);
#14652=ORIENTED_EDGE('',*,*,#10916,.F.);
#14653=ORIENTED_EDGE('',*,*,#10917,.T.);
#14654=ORIENTED_EDGE('',*,*,#10918,.T.);
#14655=ORIENTED_EDGE('',*,*,#10914,.T.);
#14656=ORIENTED_EDGE('',*,*,#10917,.F.);
#14657=ORIENTED_EDGE('',*,*,#10919,.T.);
#14658=ORIENTED_EDGE('',*,*,#10920,.F.);
#14659=ORIENTED_EDGE('',*,*,#10921,.F.);
#14660=ORIENTED_EDGE('',*,*,#10922,.F.);
#14661=ORIENTED_EDGE('',*,*,#10923,.T.);
#14662=ORIENTED_EDGE('',*,*,#10924,.T.);
#14663=ORIENTED_EDGE('',*,*,#10920,.T.);
#14664=ORIENTED_EDGE('',*,*,#10923,.F.);
#14665=ORIENTED_EDGE('',*,*,#10925,.T.);
#14666=ORIENTED_EDGE('',*,*,#10926,.F.);
#14667=ORIENTED_EDGE('',*,*,#10927,.F.);
#14668=ORIENTED_EDGE('',*,*,#10928,.F.);
#14669=ORIENTED_EDGE('',*,*,#10929,.T.);
#14670=ORIENTED_EDGE('',*,*,#10930,.T.);
#14671=ORIENTED_EDGE('',*,*,#10926,.T.);
#14672=ORIENTED_EDGE('',*,*,#10909,.T.);
#14673=ORIENTED_EDGE('',*,*,#10931,.F.);
#14674=ORIENTED_EDGE('',*,*,#10928,.T.);
#14675=ORIENTED_EDGE('',*,*,#10925,.F.);
#14676=ORIENTED_EDGE('',*,*,#10922,.T.);
#14677=ORIENTED_EDGE('',*,*,#10919,.F.);
#14678=ORIENTED_EDGE('',*,*,#10916,.T.);
#14679=ORIENTED_EDGE('',*,*,#10913,.F.);
#14680=ORIENTED_EDGE('',*,*,#10912,.F.);
#14681=ORIENTED_EDGE('',*,*,#10932,.F.);
#14682=ORIENTED_EDGE('',*,*,#10929,.F.);
#14683=ORIENTED_EDGE('',*,*,#10931,.T.);
#14684=ORIENTED_EDGE('',*,*,#10813,.T.);
#14685=ORIENTED_EDGE('',*,*,#10898,.T.);
#14686=ORIENTED_EDGE('',*,*,#10842,.T.);
#14687=ORIENTED_EDGE('',*,*,#10846,.F.);
#14688=ORIENTED_EDGE('',*,*,#10838,.T.);
#14689=ORIENTED_EDGE('',*,*,#10809,.T.);
#14690=ORIENTED_EDGE('',*,*,#10801,.T.);
#14691=ORIENTED_EDGE('',*,*,#10853,.T.);
#14692=ORIENTED_EDGE('',*,*,#10908,.T.);
#14693=ORIENTED_EDGE('',*,*,#10933,.T.);
#14694=ORIENTED_EDGE('',*,*,#10793,.T.);
#14695=ORIENTED_EDGE('',*,*,#10934,.F.);
#14696=ORIENTED_EDGE('',*,*,#10935,.T.);
#14697=ORIENTED_EDGE('',*,*,#10856,.F.);
#14698=ORIENTED_EDGE('',*,*,#10935,.F.);
#14699=ORIENTED_EDGE('',*,*,#10782,.T.);
#14700=ORIENTED_EDGE('',*,*,#10936,.T.);
#14701=ORIENTED_EDGE('',*,*,#10937,.F.);
#14702=ORIENTED_EDGE('',*,*,#10906,.F.);
#14703=ORIENTED_EDGE('',*,*,#10904,.F.);
#14704=ORIENTED_EDGE('',*,*,#10938,.T.);
#14705=ORIENTED_EDGE('',*,*,#10848,.F.);
#14706=ORIENTED_EDGE('',*,*,#10905,.F.);
#14707=ORIENTED_EDGE('',*,*,#10939,.F.);
#14708=ORIENTED_EDGE('',*,*,#10940,.F.);
#14709=ORIENTED_EDGE('',*,*,#10941,.F.);
#14710=ORIENTED_EDGE('',*,*,#10942,.F.);
#14711=ORIENTED_EDGE('',*,*,#10943,.F.);
#14712=ORIENTED_EDGE('',*,*,#10941,.T.);
#14713=ORIENTED_EDGE('',*,*,#10944,.F.);
#14714=ORIENTED_EDGE('',*,*,#10895,.F.);
#14715=ORIENTED_EDGE('',*,*,#10945,.F.);
#14716=ORIENTED_EDGE('',*,*,#10893,.F.);
#14717=ORIENTED_EDGE('',*,*,#10894,.F.);
#14718=ORIENTED_EDGE('',*,*,#10945,.T.);
#14719=ORIENTED_EDGE('',*,*,#10946,.F.);
#14720=ORIENTED_EDGE('',*,*,#10947,.F.);
#14721=ORIENTED_EDGE('',*,*,#10948,.F.);
#14722=ORIENTED_EDGE('',*,*,#10949,.F.);
#14723=ORIENTED_EDGE('',*,*,#10950,.F.);
#14724=ORIENTED_EDGE('',*,*,#10948,.T.);
#14725=ORIENTED_EDGE('',*,*,#10871,.F.);
#14726=ORIENTED_EDGE('',*,*,#10951,.T.);
#14727=ORIENTED_EDGE('',*,*,#10942,.T.);
#14728=ORIENTED_EDGE('',*,*,#10943,.T.);
#14729=ORIENTED_EDGE('',*,*,#10940,.T.);
#14730=ORIENTED_EDGE('',*,*,#10952,.T.);
#14731=ORIENTED_EDGE('',*,*,#10953,.F.);
#14732=ORIENTED_EDGE('',*,*,#10875,.F.);
#14733=ORIENTED_EDGE('',*,*,#10949,.T.);
#14734=ORIENTED_EDGE('',*,*,#10950,.T.);
#14735=ORIENTED_EDGE('',*,*,#10947,.T.);
#14736=ORIENTED_EDGE('',*,*,#10954,.T.);
#14737=ORIENTED_EDGE('',*,*,#10955,.F.);
#14738=ORIENTED_EDGE('',*,*,#10879,.F.);
#14739=ORIENTED_EDGE('',*,*,#10956,.T.);
#14740=ORIENTED_EDGE('',*,*,#10957,.T.);
#14741=ORIENTED_EDGE('',*,*,#10958,.F.);
#14742=ORIENTED_EDGE('',*,*,#10959,.F.);
#14743=ORIENTED_EDGE('',*,*,#10960,.F.);
#14744=ORIENTED_EDGE('',*,*,#10961,.F.);
#14745=ORIENTED_EDGE('',*,*,#10962,.F.);
#14746=ORIENTED_EDGE('',*,*,#10960,.T.);
#14747=ORIENTED_EDGE('',*,*,#10961,.T.);
#14748=ORIENTED_EDGE('',*,*,#10962,.T.);
#14749=ORIENTED_EDGE('',*,*,#10959,.T.);
#14750=ORIENTED_EDGE('',*,*,#10963,.T.);
#14751=ORIENTED_EDGE('',*,*,#10964,.F.);
#14752=ORIENTED_EDGE('',*,*,#10877,.F.);
#14753=ORIENTED_EDGE('',*,*,#10965,.T.);
#14754=ORIENTED_EDGE('',*,*,#10966,.T.);
#14755=ORIENTED_EDGE('',*,*,#10805,.T.);
#14756=ORIENTED_EDGE('',*,*,#10818,.T.);
#14757=ORIENTED_EDGE('',*,*,#10733,.T.);
#14758=ORIENTED_EDGE('',*,*,#10734,.T.);
#14759=ORIENTED_EDGE('',*,*,#10850,.T.);
#14760=ORIENTED_EDGE('',*,*,#10797,.T.);
#14761=ORIENTED_EDGE('',*,*,#10967,.T.);
#14762=ORIENTED_EDGE('',*,*,#10968,.T.);
#14763=ORIENTED_EDGE('',*,*,#10969,.T.);
#14764=ORIENTED_EDGE('',*,*,#10968,.F.);
#14765=ORIENTED_EDGE('',*,*,#10969,.F.);
#14766=ORIENTED_EDGE('',*,*,#10970,.F.);
#14767=ORIENTED_EDGE('',*,*,#10971,.T.);
#14768=ORIENTED_EDGE('',*,*,#10972,.T.);
#14769=ORIENTED_EDGE('',*,*,#10967,.F.);
#14770=ORIENTED_EDGE('',*,*,#10972,.F.);
#14771=ORIENTED_EDGE('',*,*,#10973,.T.);
#14772=ORIENTED_EDGE('',*,*,#10974,.T.);
#14773=ORIENTED_EDGE('',*,*,#10970,.T.);
#14774=ORIENTED_EDGE('',*,*,#10974,.F.);
#14775=ORIENTED_EDGE('',*,*,#10975,.T.);
#14776=ORIENTED_EDGE('',*,*,#10973,.F.);
#14777=ORIENTED_EDGE('',*,*,#10976,.T.);
#14778=ORIENTED_EDGE('',*,*,#10977,.T.);
#14779=ORIENTED_EDGE('',*,*,#10976,.F.);
#14780=ORIENTED_EDGE('',*,*,#10975,.F.);
#14781=ORIENTED_EDGE('',*,*,#10859,.T.);
#14782=ORIENTED_EDGE('',*,*,#10978,.F.);
#14783=ORIENTED_EDGE('',*,*,#10884,.F.);
#14784=ORIENTED_EDGE('',*,*,#10979,.T.);
#14785=ORIENTED_EDGE('',*,*,#10978,.T.);
#14786=ORIENTED_EDGE('',*,*,#10979,.F.);
#14787=ORIENTED_EDGE('',*,*,#10866,.T.);
#14788=ORIENTED_EDGE('',*,*,#10980,.F.);
#14789=ORIENTED_EDGE('',*,*,#10885,.F.);
#14790=ORIENTED_EDGE('',*,*,#10981,.T.);
#14791=ORIENTED_EDGE('',*,*,#10980,.T.);
#14792=ORIENTED_EDGE('',*,*,#10981,.F.);
#14793=ORIENTED_EDGE('',*,*,#10864,.T.);
#14794=ORIENTED_EDGE('',*,*,#10982,.F.);
#14795=ORIENTED_EDGE('',*,*,#10886,.F.);
#14796=ORIENTED_EDGE('',*,*,#10983,.T.);
#14797=ORIENTED_EDGE('',*,*,#10982,.T.);
#14798=ORIENTED_EDGE('',*,*,#10983,.F.);
#14799=ORIENTED_EDGE('',*,*,#10857,.T.);
#14800=ORIENTED_EDGE('',*,*,#10984,.F.);
#14801=ORIENTED_EDGE('',*,*,#10887,.F.);
#14802=ORIENTED_EDGE('',*,*,#10985,.T.);
#14803=ORIENTED_EDGE('',*,*,#10984,.T.);
#14804=ORIENTED_EDGE('',*,*,#10985,.F.);
#14805=ORIENTED_EDGE('',*,*,#10777,.T.);
#14806=ORIENTED_EDGE('',*,*,#10843,.F.);
#14807=ORIENTED_EDGE('',*,*,#10897,.F.);
#14808=ORIENTED_EDGE('',*,*,#10889,.F.);
#14809=ORIENTED_EDGE('',*,*,#10896,.F.);
#14810=ORIENTED_EDGE('',*,*,#10944,.T.);
#14811=ORIENTED_EDGE('',*,*,#10892,.F.);
#14812=ORIENTED_EDGE('',*,*,#10986,.F.);
#14813=ORIENTED_EDGE('',*,*,#10954,.F.);
#14814=ORIENTED_EDGE('',*,*,#10946,.T.);
#14815=ORIENTED_EDGE('',*,*,#10957,.F.);
#14816=ORIENTED_EDGE('',*,*,#10987,.F.);
#14817=ORIENTED_EDGE('',*,*,#10963,.F.);
#14818=ORIENTED_EDGE('',*,*,#10958,.T.);
#14819=ORIENTED_EDGE('',*,*,#10966,.F.);
#14820=ORIENTED_EDGE('',*,*,#10988,.F.);
#14821=ORIENTED_EDGE('',*,*,#10952,.F.);
#14822=ORIENTED_EDGE('',*,*,#10939,.T.);
#14823=ORIENTED_EDGE('',*,*,#10951,.F.);
#14824=ORIENTED_EDGE('',*,*,#10870,.F.);
#14825=ORIENTED_EDGE('',*,*,#10873,.F.);
#14826=ORIENTED_EDGE('',*,*,#10936,.F.);
#14827=ORIENTED_EDGE('',*,*,#10781,.T.);
#14828=ORIENTED_EDGE('',*,*,#10785,.T.);
#14829=ORIENTED_EDGE('',*,*,#10849,.F.);
#14830=ORIENTED_EDGE('',*,*,#10938,.F.);
#14831=ORIENTED_EDGE('',*,*,#10903,.F.);
#14832=ORIENTED_EDGE('',*,*,#10814,.T.);
#14833=ORIENTED_EDGE('',*,*,#10927,.T.);
#14834=ORIENTED_EDGE('',*,*,#10930,.F.);
#14835=ORIENTED_EDGE('',*,*,#10932,.T.);
#14836=ORIENTED_EDGE('',*,*,#10911,.F.);
#14837=ORIENTED_EDGE('',*,*,#10915,.T.);
#14838=ORIENTED_EDGE('',*,*,#10918,.F.);
#14839=ORIENTED_EDGE('',*,*,#10921,.T.);
#14840=ORIENTED_EDGE('',*,*,#10924,.F.);
#14841=ORIENTED_EDGE('',*,*,#10971,.F.);
#14842=ORIENTED_EDGE('',*,*,#10989,.F.);
#14843=ORIENTED_EDGE('',*,*,#10990,.T.);
#14844=ORIENTED_EDGE('',*,*,#10991,.T.);
#14845=ORIENTED_EDGE('',*,*,#10990,.F.);
#14846=ORIENTED_EDGE('',*,*,#10991,.F.);
#14847=ORIENTED_EDGE('',*,*,#10934,.T.);
#14848=ORIENTED_EDGE('',*,*,#10977,.F.);
#14849=ORIENTED_EDGE('',*,*,#10989,.T.);
#14850=ORIENTED_EDGE('',*,*,#10880,.F.);
#14851=ORIENTED_EDGE('',*,*,#10955,.T.);
#14852=ORIENTED_EDGE('',*,*,#10986,.T.);
#14853=ORIENTED_EDGE('',*,*,#10891,.F.);
#14854=ORIENTED_EDGE('',*,*,#10878,.F.);
#14855=ORIENTED_EDGE('',*,*,#10964,.T.);
#14856=ORIENTED_EDGE('',*,*,#10987,.T.);
#14857=ORIENTED_EDGE('',*,*,#10956,.F.);
#14858=ORIENTED_EDGE('',*,*,#10876,.F.);
#14859=ORIENTED_EDGE('',*,*,#10953,.T.);
#14860=ORIENTED_EDGE('',*,*,#10988,.T.);
#14861=ORIENTED_EDGE('',*,*,#10965,.F.);
#14862=ORIENTED_EDGE('',*,*,#10794,.T.);
#14863=ORIENTED_EDGE('',*,*,#10933,.F.);
#14864=ORIENTED_EDGE('',*,*,#10907,.T.);
#14865=ORIENTED_EDGE('',*,*,#10937,.T.);
#14866=ORIENTED_EDGE('',*,*,#10872,.T.);
#14867=ORIENTED_EDGE('',*,*,#10789,.T.);
#18789=ADVANCED_FACE('',(#5073),#719,.F.);
#18790=ADVANCED_FACE('',(#5074),#4430,.T.);
#18791=ADVANCED_FACE('',(#5075),#4431,.T.);
#18792=ADVANCED_FACE('',(#5076),#4432,.T.);
#18793=ADVANCED_FACE('',(#5077),#720,.F.);
#18794=ADVANCED_FACE('',(#5078),#4433,.T.);
#18795=ADVANCED_FACE('',(#5079),#4434,.T.);
#18796=ADVANCED_FACE('',(#5080),#4435,.T.);
#18797=ADVANCED_FACE('',(#5081),#721,.F.);
#18798=ADVANCED_FACE('',(#5082),#4436,.T.);
#18799=ADVANCED_FACE('',(#5083),#4437,.T.);
#18800=ADVANCED_FACE('',(#5084),#722,.F.);
#18801=ADVANCED_FACE('',(#5085),#723,.F.);
#18802=ADVANCED_FACE('',(#5086),#724,.F.);
#18803=ADVANCED_FACE('',(#5087),#725,.F.);
#18804=ADVANCED_FACE('',(#5088),#4438,.T.);
#18805=ADVANCED_FACE('',(#5089),#4439,.T.);
#18806=ADVANCED_FACE('',(#5090),#4440,.T.);
#18807=ADVANCED_FACE('',(#5091),#4441,.T.);
#18808=ADVANCED_FACE('',(#5092),#726,.F.);
#18809=ADVANCED_FACE('',(#5093),#727,.F.);
#18810=ADVANCED_FACE('',(#5094),#728,.T.);
#18811=ADVANCED_FACE('',(#5095),#174,.F.);
#18812=ADVANCED_FACE('',(#5096),#729,.T.);
#18813=ADVANCED_FACE('',(#5097),#730,.T.);
#18814=ADVANCED_FACE('',(#5098),#175,.F.);
#18815=ADVANCED_FACE('',(#5099),#731,.T.);
#18816=ADVANCED_FACE('',(#5100),#732,.T.);
#18817=ADVANCED_FACE('',(#5101),#176,.F.);
#18818=ADVANCED_FACE('',(#5102),#733,.T.);
#18819=ADVANCED_FACE('',(#5103),#734,.T.);
#18820=ADVANCED_FACE('',(#5104),#735,.T.);
#18821=ADVANCED_FACE('',(#5105),#736,.T.);
#18822=ADVANCED_FACE('',(#5106,#503),#737,.T.);
#18823=ADVANCED_FACE('',(#5107),#4442,.F.);
#18824=ADVANCED_FACE('',(#5108),#4443,.F.);
#18825=ADVANCED_FACE('',(#5109),#177,.F.);
#18826=ADVANCED_FACE('',(#5110),#4444,.F.);
#18827=ADVANCED_FACE('',(#5111),#4445,.F.);
#18828=ADVANCED_FACE('',(#5112),#4446,.T.);
#18829=ADVANCED_FACE('',(#5113),#738,.F.);
#18830=ADVANCED_FACE('',(#5114,#504,#505,#506,#507),#739,.F.);
#18831=ADVANCED_FACE('',(#5115),#4447,.T.);
#18832=ADVANCED_FACE('',(#5116),#740,.F.);
#18833=ADVANCED_FACE('',(#5117),#741,.F.);
#18834=ADVANCED_FACE('',(#5118),#742,.T.);
#18835=ADVANCED_FACE('',(#5119),#743,.T.);
#18836=ADVANCED_FACE('',(#5120),#744,.T.);
#18837=ADVANCED_FACE('',(#5121),#745,.T.);
#18838=ADVANCED_FACE('',(#5122),#746,.T.);
#18839=ADVANCED_FACE('',(#5123),#4448,.F.);
#18840=ADVANCED_FACE('',(#5124),#747,.F.);
#18841=ADVANCED_FACE('',(#5125),#4449,.F.);
#18842=ADVANCED_FACE('',(#5126),#748,.F.);
#18843=ADVANCED_FACE('',(#5127),#4450,.F.);
#18844=ADVANCED_FACE('',(#5128),#749,.F.);
#18845=ADVANCED_FACE('',(#5129),#4451,.F.);
#18846=ADVANCED_FACE('',(#5130),#750,.F.);
#18847=ADVANCED_FACE('',(#5131),#751,.F.);
#18848=ADVANCED_FACE('',(#5132),#752,.T.);
#18849=ADVANCED_FACE('',(#5133),#753,.T.);
#18850=ADVANCED_FACE('',(#5134),#4452,.F.);
#18851=ADVANCED_FACE('',(#5135),#754,.T.);
#18852=ADVANCED_FACE('',(#5136),#755,.T.);
#18853=ADVANCED_FACE('',(#5137),#4453,.T.);
#18854=ADVANCED_FACE('',(#5138),#756,.T.);
#18855=ADVANCED_FACE('',(#5139),#4454,.T.);
#18856=ADVANCED_FACE('',(#5140),#757,.T.);
#18857=ADVANCED_FACE('',(#5141),#4455,.T.);
#18858=ADVANCED_FACE('',(#5142),#758,.T.);
#18859=ADVANCED_FACE('',(#5143),#759,.F.);
#18860=ADVANCED_FACE('',(#5144),#760,.F.);
#18861=ADVANCED_FACE('',(#5145),#4456,.T.);
#18862=ADVANCED_FACE('',(#5146),#761,.T.);
#18863=ADVANCED_FACE('',(#5147),#762,.F.);
#18864=ADVANCED_FACE('',(#5148),#763,.T.);
#18865=ADVANCED_FACE('',(#5149),#178,.T.);
#18866=ADVANCED_FACE('',(#5150,#508),#764,.T.);
#18867=ADVANCED_FACE('',(#5151),#4457,.T.);
#18868=ADVANCED_FACE('',(#5152),#179,.F.);
#18869=ADVANCED_FACE('',(#5153),#4458,.F.);
#18870=ADVANCED_FACE('',(#5154,#509),#765,.T.);
#18871=ADVANCED_FACE('',(#5155),#4459,.F.);
#18872=ADVANCED_FACE('',(#5156,#510),#766,.T.);
#18873=ADVANCED_FACE('',(#5157),#4460,.F.);
#18874=ADVANCED_FACE('',(#5158,#511),#767,.T.);
#18875=ADVANCED_FACE('',(#5159),#4461,.F.);
#18876=ADVANCED_FACE('',(#5160,#512),#768,.T.);
#18877=ADVANCED_FACE('',(#5161),#4462,.F.);
#18878=ADVANCED_FACE('',(#5162,#513,#514),#769,.T.);
#18879=ADVANCED_FACE('',(#5163),#4463,.F.);
#18880=ADVANCED_FACE('',(#5164,#515),#770,.T.);
#18881=ADVANCED_FACE('',(#5165,#516),#771,.T.);
#18882=ADVANCED_FACE('',(#5166),#772,.F.);
#18883=ADVANCED_FACE('',(#5167),#773,.F.);
#18884=ADVANCED_FACE('',(#5168),#774,.F.);
#18885=ADVANCED_FACE('',(#5169),#775,.T.);
#19559=CLOSED_SHELL('',(#18789,#18790,#18791,#18792,#18793,#18794,#18795,
#18796,#18797,#18798,#18799,#18800,#18801,#18802,#18803,#18804,#18805,#18806,
#18807,#18808,#18809,#18810,#18811,#18812,#18813,#18814,#18815,#18816,#18817,
#18818,#18819,#18820,#18821,#18822,#18823,#18824,#18825,#18826,#18827,#18828,
#18829,#18830,#18831,#18832,#18833,#18834,#18835,#18836,#18837,#18838,#18839,
#18840,#18841,#18842,#18843,#18844,#18845,#18846,#18847,#18848,#18849,#18850,
#18851,#18852,#18853,#18854,#18855,#18856,#18857,#18858,#18859,#18860,#18861,
#18862,#18863,#18864,#18865,#18866,#18867,#18868,#18869,#18870,#18871,#18872,
#18873,#18874,#18875,#18876,#18877,#18878,#18879,#18880,#18881,#18882,#18883,
#18884,#18885));
#20591=AXIS2_PLACEMENT_3D('',#30302,#23933,#23934);
#20592=AXIS2_PLACEMENT_3D('',#30303,#23935,#23936);
#20593=AXIS2_PLACEMENT_3D('',#30312,#23941,#23942);
#20594=AXIS2_PLACEMENT_3D('',#30314,#23943,#23944);
#20595=AXIS2_PLACEMENT_3D('',#30316,#23945,#23946);
#20596=AXIS2_PLACEMENT_3D('',#30319,#23948,#23949);
#20597=AXIS2_PLACEMENT_3D('',#30320,#23950,#23951);
#20598=AXIS2_PLACEMENT_3D('',#30322,#23952,#23953);
#20599=AXIS2_PLACEMENT_3D('',#30324,#23954,#23955);
#20600=AXIS2_PLACEMENT_3D('',#30328,#23957,#23958);
#20601=AXIS2_PLACEMENT_3D('',#30330,#23959,#23960);
#20602=AXIS2_PLACEMENT_3D('',#30338,#23961,#23962);
#20603=AXIS2_PLACEMENT_3D('',#30339,#23963,#23964);
#20604=AXIS2_PLACEMENT_3D('',#30341,#23965,#23966);
#20605=AXIS2_PLACEMENT_3D('',#30343,#23967,#23968);
#20606=AXIS2_PLACEMENT_3D('',#30346,#23970,#23971);
#20607=AXIS2_PLACEMENT_3D('',#30347,#23972,#23973);
#20608=AXIS2_PLACEMENT_3D('',#30353,#23977,#23978);
#20609=AXIS2_PLACEMENT_3D('',#30355,#23979,#23980);
#20610=AXIS2_PLACEMENT_3D('',#30357,#23981,#23982);
#20611=AXIS2_PLACEMENT_3D('',#30360,#23984,#23985);
#20612=AXIS2_PLACEMENT_3D('',#30361,#23986,#23987);
#20613=AXIS2_PLACEMENT_3D('',#30363,#23988,#23989);
#20614=AXIS2_PLACEMENT_3D('',#30365,#23990,#23991);
#20615=AXIS2_PLACEMENT_3D('',#30369,#23993,#23994);
#20616=AXIS2_PLACEMENT_3D('',#30371,#23995,#23996);
#20617=AXIS2_PLACEMENT_3D('',#30379,#23997,#23998);
#20618=AXIS2_PLACEMENT_3D('',#30380,#23999,#24000);
#20619=AXIS2_PLACEMENT_3D('',#30382,#24001,#24002);
#20620=AXIS2_PLACEMENT_3D('',#30384,#24003,#24004);
#20621=AXIS2_PLACEMENT_3D('',#30387,#24006,#24007);
#20622=AXIS2_PLACEMENT_3D('',#30388,#24008,#24009);
#20623=AXIS2_PLACEMENT_3D('',#30394,#24013,#24014);
#20624=AXIS2_PLACEMENT_3D('',#30396,#24015,#24016);
#20625=AXIS2_PLACEMENT_3D('',#30398,#24017,#24018);
#20626=AXIS2_PLACEMENT_3D('',#30401,#24020,#24021);
#20627=AXIS2_PLACEMENT_3D('',#30402,#24022,#24023);
#20628=AXIS2_PLACEMENT_3D('',#30404,#24024,#24025);
#20629=AXIS2_PLACEMENT_3D('',#30406,#24026,#24027);
#20630=AXIS2_PLACEMENT_3D('',#30410,#24029,#24030);
#20631=AXIS2_PLACEMENT_3D('',#30412,#24031,#24032);
#20632=AXIS2_PLACEMENT_3D('',#30420,#24033,#24034);
#20633=AXIS2_PLACEMENT_3D('',#30421,#24035,#24036);
#20634=AXIS2_PLACEMENT_3D('',#30430,#24041,#24042);
#20635=AXIS2_PLACEMENT_3D('',#30439,#24047,#24048);
#20636=AXIS2_PLACEMENT_3D('',#30447,#24053,#24054);
#20637=AXIS2_PLACEMENT_3D('',#30456,#24059,#24060);
#20638=AXIS2_PLACEMENT_3D('',#30459,#24061,#24062);
#20639=AXIS2_PLACEMENT_3D('',#30460,#24063,#24064);
#20640=AXIS2_PLACEMENT_3D('',#30462,#24065,#24066);
#20641=AXIS2_PLACEMENT_3D('',#30464,#24068,#24069);
#20642=AXIS2_PLACEMENT_3D('',#30467,#24070,#24071);
#20643=AXIS2_PLACEMENT_3D('',#30469,#24072,#24073);
#20644=AXIS2_PLACEMENT_3D('',#30478,#24074,#24075);
#20645=AXIS2_PLACEMENT_3D('',#30479,#24076,#24077);
#20646=AXIS2_PLACEMENT_3D('',#30481,#24078,#24079);
#20647=AXIS2_PLACEMENT_3D('',#30483,#24081,#24082);
#20648=AXIS2_PLACEMENT_3D('',#30485,#24083,#24084);
#20649=AXIS2_PLACEMENT_3D('',#30486,#24085,#24086);
#20650=AXIS2_PLACEMENT_3D('',#30487,#24087,#24088);
#20651=AXIS2_PLACEMENT_3D('',#30488,#24089,#24090);
#20652=AXIS2_PLACEMENT_3D('',#30490,#24091,#24092);
#20653=AXIS2_PLACEMENT_3D('',#30494,#24094,#24095);
#20654=AXIS2_PLACEMENT_3D('',#30495,#24096,#24097);
#20655=AXIS2_PLACEMENT_3D('',#30496,#24098,#24099);
#20656=AXIS2_PLACEMENT_3D('',#30502,#24103,#24104);
#20657=AXIS2_PLACEMENT_3D('',#30510,#24109,#24110);
#20658=AXIS2_PLACEMENT_3D('',#30512,#24112,#24113);
#20659=AXIS2_PLACEMENT_3D('',#30515,#24114,#24115);
#20660=AXIS2_PLACEMENT_3D('',#30518,#24117,#24118);
#20661=AXIS2_PLACEMENT_3D('',#30519,#24119,#24120);
#20662=AXIS2_PLACEMENT_3D('',#30520,#24121,#24122);
#20663=AXIS2_PLACEMENT_3D('',#30521,#24123,#24124);
#20664=AXIS2_PLACEMENT_3D('',#30523,#24126,#24127);
#20665=AXIS2_PLACEMENT_3D('',#30525,#24129,#24130);
#20666=AXIS2_PLACEMENT_3D('',#30528,#24131,#24132);
#20667=AXIS2_PLACEMENT_3D('',#30531,#24134,#24135);
#20668=AXIS2_PLACEMENT_3D('',#30532,#24136,#24137);
#20669=AXIS2_PLACEMENT_3D('',#30533,#24138,#24139);
#20670=AXIS2_PLACEMENT_3D('',#30534,#24140,#24141);
#20671=AXIS2_PLACEMENT_3D('',#30536,#24143,#24144);
#20672=AXIS2_PLACEMENT_3D('',#30538,#24146,#24147);
#20673=AXIS2_PLACEMENT_3D('',#30541,#24148,#24149);
#20674=AXIS2_PLACEMENT_3D('',#30544,#24151,#24152);
#20675=AXIS2_PLACEMENT_3D('',#30545,#24153,#24154);
#20676=AXIS2_PLACEMENT_3D('',#30546,#24155,#24156);
#20677=AXIS2_PLACEMENT_3D('',#30547,#24157,#24158);
#20678=AXIS2_PLACEMENT_3D('',#30553,#24162,#24163);
#20679=AXIS2_PLACEMENT_3D('',#30559,#24167,#24168);
#20680=AXIS2_PLACEMENT_3D('',#30564,#24172,#24173);
#20681=AXIS2_PLACEMENT_3D('',#30570,#24177,#24178);
#20682=AXIS2_PLACEMENT_3D('',#30578,#24183,#24184);
#20683=AXIS2_PLACEMENT_3D('',#30579,#24185,#24186);
#20684=AXIS2_PLACEMENT_3D('',#30581,#24187,#24188);
#20685=AXIS2_PLACEMENT_3D('',#30582,#24189,#24190);
#20686=AXIS2_PLACEMENT_3D('',#30584,#24191,#24192);
#20687=AXIS2_PLACEMENT_3D('',#30586,#24194,#24195);
#20688=AXIS2_PLACEMENT_3D('',#30588,#24196,#24197);
#20689=AXIS2_PLACEMENT_3D('',#30590,#24199,#24200);
#20690=AXIS2_PLACEMENT_3D('',#30593,#24201,#24202);
#20691=AXIS2_PLACEMENT_3D('',#30595,#24204,#24205);
#20692=AXIS2_PLACEMENT_3D('',#30596,#24206,#24207);
#20693=AXIS2_PLACEMENT_3D('',#30598,#24208,#24209);
#20694=AXIS2_PLACEMENT_3D('',#30600,#24211,#24212);
#20695=AXIS2_PLACEMENT_3D('',#30602,#24213,#24214);
#20696=AXIS2_PLACEMENT_3D('',#30604,#24216,#24217);
#20697=AXIS2_PLACEMENT_3D('',#30607,#24218,#24219);
#20698=AXIS2_PLACEMENT_3D('',#30611,#24221,#24222);
#20699=AXIS2_PLACEMENT_3D('',#30613,#24224,#24225);
#20700=AXIS2_PLACEMENT_3D('',#30618,#24229,#24230);
#20701=AXIS2_PLACEMENT_3D('',#30634,#24238,#24239);
#20702=AXIS2_PLACEMENT_3D('',#30637,#24241,#24242);
#20703=AXIS2_PLACEMENT_3D('',#30639,#24243,#24244);
#20704=AXIS2_PLACEMENT_3D('',#30641,#24245,#24246);
#20705=AXIS2_PLACEMENT_3D('',#30643,#24247,#24248);
#20706=AXIS2_PLACEMENT_3D('',#30644,#24249,#24250);
#20707=AXIS2_PLACEMENT_3D('',#30648,#24252,#24253);
#20708=AXIS2_PLACEMENT_3D('',#30650,#24255,#24256);
#20709=AXIS2_PLACEMENT_3D('',#30662,#24263,#24264);
#20710=AXIS2_PLACEMENT_3D('',#30665,#24267,#24268);
#20711=AXIS2_PLACEMENT_3D('',#30668,#24271,#24272);
#20712=AXIS2_PLACEMENT_3D('',#30672,#24275,#24276);
#20713=AXIS2_PLACEMENT_3D('',#30676,#24279,#24280);
#20714=AXIS2_PLACEMENT_3D('',#30678,#24282,#24283);
#20715=AXIS2_PLACEMENT_3D('',#30684,#24287,#24288);
#20716=AXIS2_PLACEMENT_3D('',#30687,#24289,#24290);
#20717=AXIS2_PLACEMENT_3D('',#30691,#24292,#24293);
#20718=AXIS2_PLACEMENT_3D('',#30693,#24295,#24296);
#20719=AXIS2_PLACEMENT_3D('',#30699,#24300,#24301);
#20720=AXIS2_PLACEMENT_3D('',#30701,#24302,#24303);
#20721=AXIS2_PLACEMENT_3D('',#30704,#24305,#24306);
#20722=AXIS2_PLACEMENT_3D('',#30705,#24307,#24308);
#20723=AXIS2_PLACEMENT_3D('',#30711,#24312,#24313);
#20724=AXIS2_PLACEMENT_3D('',#30713,#24314,#24315);
#20725=AXIS2_PLACEMENT_3D('',#30716,#24317,#24318);
#20726=AXIS2_PLACEMENT_3D('',#30717,#24319,#24320);
#20727=AXIS2_PLACEMENT_3D('',#30723,#24324,#24325);
#20728=AXIS2_PLACEMENT_3D('',#30725,#24326,#24327);
#20729=AXIS2_PLACEMENT_3D('',#30728,#24329,#24330);
#20730=AXIS2_PLACEMENT_3D('',#30729,#24331,#24332);
#20731=AXIS2_PLACEMENT_3D('',#30731,#24334,#24335);
#20732=AXIS2_PLACEMENT_3D('',#30733,#24337,#24338);
#20733=AXIS2_PLACEMENT_3D('',#30734,#24339,#24340);
#20734=AXIS2_PLACEMENT_3D('',#30736,#24342,#24343);
#20735=AXIS2_PLACEMENT_3D('',#30738,#24344,#24345);
#20736=AXIS2_PLACEMENT_3D('',#30740,#24347,#24348);
#20737=AXIS2_PLACEMENT_3D('',#30743,#24351,#24352);
#20738=AXIS2_PLACEMENT_3D('',#30745,#24354,#24355);
#20739=AXIS2_PLACEMENT_3D('',#30748,#24356,#24357);
#20740=AXIS2_PLACEMENT_3D('',#30752,#24359,#24360);
#20741=AXIS2_PLACEMENT_3D('',#30754,#24362,#24363);
#20742=AXIS2_PLACEMENT_3D('',#30756,#24365,#24366);
#20743=AXIS2_PLACEMENT_3D('',#30757,#24367,#24368);
#20744=AXIS2_PLACEMENT_3D('',#30758,#24369,#24370);
#20745=AXIS2_PLACEMENT_3D('',#30759,#24371,#24372);
#20746=AXIS2_PLACEMENT_3D('',#30760,#24373,#24374);
#20747=AXIS2_PLACEMENT_3D('',#30763,#24375,#24376);
#20748=AXIS2_PLACEMENT_3D('',#30767,#24378,#24379);
#20749=AXIS2_PLACEMENT_3D('',#30769,#24381,#24382);
#20750=AXIS2_PLACEMENT_3D('',#30771,#24384,#24385);
#20751=AXIS2_PLACEMENT_3D('',#30776,#24389,#24390);
#20752=AXIS2_PLACEMENT_3D('',#30783,#24395,#24396);
#20753=AXIS2_PLACEMENT_3D('',#30786,#24397,#24398);
#20754=AXIS2_PLACEMENT_3D('',#30790,#24400,#24401);
#20755=AXIS2_PLACEMENT_3D('',#30792,#24403,#24404);
#20756=AXIS2_PLACEMENT_3D('',#30794,#24406,#24407);
#20757=AXIS2_PLACEMENT_3D('',#30801,#24412,#24413);
#20758=AXIS2_PLACEMENT_3D('',#30802,#24414,#24415);
#20759=AXIS2_PLACEMENT_3D('',#30804,#24416,#24417);
#20760=AXIS2_PLACEMENT_3D('',#30807,#24419,#24420);
#20761=AXIS2_PLACEMENT_3D('',#30808,#24421,#24422);
#20762=AXIS2_PLACEMENT_3D('',#30810,#24423,#24424);
#20763=AXIS2_PLACEMENT_3D('',#30811,#24425,#24426);
#20764=AXIS2_PLACEMENT_3D('',#30813,#24427,#24428);
#20765=AXIS2_PLACEMENT_3D('',#30815,#24430,#24431);
#20766=AXIS2_PLACEMENT_3D('',#30818,#24432,#24433);
#20767=AXIS2_PLACEMENT_3D('',#30820,#24435,#24436);
#20768=AXIS2_PLACEMENT_3D('',#30821,#24437,#24438);
#20769=AXIS2_PLACEMENT_3D('',#30824,#24440,#24441);
#20770=AXIS2_PLACEMENT_3D('',#30825,#24442,#24443);
#20771=AXIS2_PLACEMENT_3D('',#30827,#24444,#24445);
#20772=AXIS2_PLACEMENT_3D('',#30828,#24446,#24447);
#20773=AXIS2_PLACEMENT_3D('',#30830,#24449,#24450);
#20774=AXIS2_PLACEMENT_3D('',#30832,#24451,#24452);
#20775=AXIS2_PLACEMENT_3D('',#30833,#24453,#24454);
#20776=AXIS2_PLACEMENT_3D('',#30835,#24456,#24457);
#20777=AXIS2_PLACEMENT_3D('',#30837,#24458,#24459);
#20778=AXIS2_PLACEMENT_3D('',#30838,#24460,#24461);
#20779=AXIS2_PLACEMENT_3D('',#30840,#24463,#24464);
#20780=AXIS2_PLACEMENT_3D('',#30842,#24465,#24466);
#20781=AXIS2_PLACEMENT_3D('',#30843,#24467,#24468);
#20782=AXIS2_PLACEMENT_3D('',#30845,#24470,#24471);
#20783=AXIS2_PLACEMENT_3D('',#30849,#24475,#24476);
#20784=AXIS2_PLACEMENT_3D('',#30851,#24477,#24478);
#20785=AXIS2_PLACEMENT_3D('',#30854,#24480,#24481);
#20786=AXIS2_PLACEMENT_3D('',#30855,#24482,#24483);
#20787=AXIS2_PLACEMENT_3D('',#30856,#24484,#24485);
#20788=AXIS2_PLACEMENT_3D('',#30857,#24486,#24487);
#20789=AXIS2_PLACEMENT_3D('',#30858,#24488,#24489);
#20790=AXIS2_PLACEMENT_3D('',#30859,#24490,#24491);
#20791=AXIS2_PLACEMENT_3D('',#30860,#24492,#24493);
#23933=DIRECTION('axis',(0.,0.,1.));
#23934=DIRECTION('refdir',(1.,0.,0.));
#23935=DIRECTION('center_axis',(-4.64905891561784E-16,0.,-1.));
#23936=DIRECTION('ref_axis',(1.,2.80259692864963E-45,-4.64905891561784E-16));
#23937=DIRECTION('',(-1.,1.13620248180482E-13,4.64905891561784E-16));
#23938=DIRECTION('',(0.,-1.,0.));
#23939=DIRECTION('',(1.,6.02124417213198E-17,-4.64905891561784E-16));
#23940=DIRECTION('',(0.,-1.,0.));
#23941=DIRECTION('center_axis',(0.,-1.,0.));
#23942=DIRECTION('ref_axis',(5.06308189820828E-12,0.,1.));
#23943=DIRECTION('center_axis',(-1.51811166660813E-15,-0.0174524064372836,
0.999847695156391));
#23944=DIRECTION('ref_axis',(8.83629631127843E-14,0.999847695156391,0.0174524064372836));
#23945=DIRECTION('center_axis',(-6.02124417213198E-17,1.,-2.60927675461843E-32));
#23946=DIRECTION('ref_axis',(5.06308189820828E-12,0.,1.));
#23947=DIRECTION('',(0.,-1.,0.));
#23948=DIRECTION('center_axis',(-1.02201073032319E-15,-0.713250449154181,
0.700909264299851));
#23949=DIRECTION('ref_axis',(3.61124543800146E-12,0.700909264299851,0.713250449154181));
#23950=DIRECTION('center_axis',(0.,-1.,0.));
#23951=DIRECTION('ref_axis',(-0.560568426943144,0.,0.828108108108168));
#23952=DIRECTION('center_axis',(-1.02201073032319E-15,-0.713250449154181,
0.700909264299851));
#23953=DIRECTION('ref_axis',(-1.0085471152714E-15,0.700909264299851,0.713250449154181));
#23954=DIRECTION('center_axis',(-6.02124417213198E-17,1.,-2.60927675461843E-32));
#23955=DIRECTION('ref_axis',(-0.560568426943144,0.,0.828108108108168));
#23956=DIRECTION('',(0.,-1.,0.));
#23957=DIRECTION('center_axis',(-0.700909264299851,-0.713250449154181,-1.06495728142559E-15));
#23958=DIRECTION('ref_axis',(-0.713250449154181,0.700909264299851,-1.19764969938479E-15));
#23959=DIRECTION('center_axis',(6.02124417213198E-17,-1.,2.60927675461843E-32));
#23960=DIRECTION('ref_axis',(-0.560568426943144,0.,0.828108108108168));
#23961=DIRECTION('center_axis',(6.02124417213198E-17,-1.,2.60927675461843E-32));
#23962=DIRECTION('ref_axis',(-0.560568426943144,0.,0.828108108108168));
#23963=DIRECTION('center_axis',(0.,-1.,0.));
#23964=DIRECTION('ref_axis',(-0.828108108108883,0.,0.560568426942087));
#23965=DIRECTION('center_axis',(-0.700909264299851,-0.713250449154181,-1.06495728142559E-15));
#23966=DIRECTION('ref_axis',(-0.713250449154181,0.700909264299851,-1.0888172225833E-15));
#23967=DIRECTION('center_axis',(-6.02124417213198E-17,1.,-2.60927675461843E-32));
#23968=DIRECTION('ref_axis',(-0.828108108108883,0.,0.560568426942087));
#23969=DIRECTION('',(0.,-1.,0.));
#23970=DIRECTION('center_axis',(-0.999847695156391,-0.0174524064372837,
-1.51916251861363E-15));
#23971=DIRECTION('ref_axis',(-0.0174524064372837,0.999847695156391,-2.66420872597733E-17));
#23972=DIRECTION('center_axis',(1.,0.,-1.22327594243755E-16));
#23973=DIRECTION('ref_axis',(1.22327594243755E-16,5.79319727271681E-31,
1.));
#23974=DIRECTION('',(-1.22327594243755E-16,9.40541631133221E-14,-1.));
#23975=DIRECTION('',(1.22327594243755E-16,3.34584106854956E-32,1.));
#23976=DIRECTION('',(0.,-1.,0.));
#23977=DIRECTION('center_axis',(0.,-1.,0.));
#23978=DIRECTION('ref_axis',(-1.,0.,5.0097911930254E-12));
#23979=DIRECTION('center_axis',(-0.999847695156391,-0.0174524064372837,
-1.51916251861363E-15));
#23980=DIRECTION('ref_axis',(-0.0174524064372837,0.999847695156391,8.74329120666037E-14));
#23981=DIRECTION('center_axis',(-6.02124417213198E-17,1.,-2.60927675461843E-32));
#23982=DIRECTION('ref_axis',(-1.,0.,5.0097911930254E-12));
#23983=DIRECTION('',(0.,-1.,0.));
#23984=DIRECTION('center_axis',(-0.700909264299851,-0.713250449154181,-1.06495728142559E-15));
#23985=DIRECTION('ref_axis',(-0.713250449154181,0.700909264299851,3.57323581859403E-12));
#23986=DIRECTION('center_axis',(0.,-1.,0.));
#23987=DIRECTION('ref_axis',(-0.828108108107798,0.,-0.56056842694369));
#23988=DIRECTION('center_axis',(-0.700909264299851,-0.713250449154181,-1.06495728142559E-15));
#23989=DIRECTION('ref_axis',(-0.713250449154181,0.700909264299851,-1.19764969938473E-15));
#23990=DIRECTION('center_axis',(-6.02124417213198E-17,1.,-2.60927675461843E-32));
#23991=DIRECTION('ref_axis',(-0.828108108107798,0.,-0.56056842694369));
#23992=DIRECTION('',(0.,-1.,0.));
#23993=DIRECTION('center_axis',(1.10790383252799E-15,-0.713250449154181,
-0.700909264299851));
#23994=DIRECTION('ref_axis',(1.19764969938473E-15,0.700909264299851,-0.713250449154181));
#23995=DIRECTION('center_axis',(6.02124417213198E-17,-1.,2.60927675461843E-32));
#23996=DIRECTION('ref_axis',(-0.828108108107798,0.,-0.56056842694369));
#23997=DIRECTION('center_axis',(6.02124417213198E-17,-1.,2.60927675461843E-32));
#23998=DIRECTION('ref_axis',(-0.828108108107798,0.,-0.56056842694369));
#23999=DIRECTION('center_axis',(0.,-1.,0.));
#24000=DIRECTION('ref_axis',(-0.560568426942121,0.,-0.82810810810886));
#24001=DIRECTION('center_axis',(1.10790383252799E-15,-0.713250449154181,
-0.700909264299851));
#24002=DIRECTION('ref_axis',(1.0888172225922E-15,0.700909264299851,-0.713250449154181));
#24003=DIRECTION('center_axis',(-6.02124417213198E-17,1.,-2.60927675461843E-32));
#24004=DIRECTION('ref_axis',(-0.560568426942121,0.,-0.82810810810886));
#24005=DIRECTION('',(0.,-1.,0.));
#24006=DIRECTION('center_axis',(1.52021337061914E-15,-0.0174524064372836,
-0.999847695156391));
#24007=DIRECTION('ref_axis',(2.66420872599909E-17,0.999847695156391,-0.0174524064372836));
#24008=DIRECTION('center_axis',(8.71984094268636E-13,0.,1.));
#24009=DIRECTION('ref_axis',(-1.,-2.54388977262688E-34,8.71984094268636E-13));
#24010=DIRECTION('',(1.,5.00430415356568E-11,-8.71984094268635E-13));
#24011=DIRECTION('',(-1.,-6.02124417213198E-17,8.71984094268636E-13));
#24012=DIRECTION('',(0.,-1.,0.));
#24013=DIRECTION('center_axis',(0.,-1.,0.));
#24014=DIRECTION('ref_axis',(-4.92541424309684E-12,0.,-1.));
#24015=DIRECTION('center_axis',(1.52021337061914E-15,-0.0174524064372836,
-0.999847695156391));
#24016=DIRECTION('ref_axis',(-8.59603312425117E-14,0.999847695156391,-0.0174524064372836));
#24017=DIRECTION('center_axis',(-6.02124417213198E-17,1.,-2.60927675461843E-32));
#24018=DIRECTION('ref_axis',(-4.92541424309684E-12,0.,-1.));
#24019=DIRECTION('',(0.,-1.,0.));
#24020=DIRECTION('center_axis',(1.10790383252799E-15,-0.713250449154181,
-0.700909264299851));
#24021=DIRECTION('ref_axis',(-3.51305392115922E-12,0.700909264299851,-0.713250449154181));
#24022=DIRECTION('center_axis',(0.,-1.,0.));
#24023=DIRECTION('ref_axis',(0.560568426943322,0.,-0.828108108108047));
#24024=DIRECTION('center_axis',(1.10790383252799E-15,-0.713250449154181,
-0.700909264299851));
#24025=DIRECTION('ref_axis',(1.13461550468027E-15,0.700909264299851,-0.713250449154181));
#24026=DIRECTION('center_axis',(-6.02124417213198E-17,1.,-2.60927675461843E-32));
#24027=DIRECTION('ref_axis',(0.560568426943322,0.,-0.828108108108047));
#24028=DIRECTION('',(0.,-1.,0.));
#24029=DIRECTION('center_axis',(0.700909264299845,-0.713250449154187,1.06495728142558E-15));
#24030=DIRECTION('ref_axis',(0.713250449154187,0.700909264299845,1.00854711527136E-15));
#24031=DIRECTION('center_axis',(6.02124417213198E-17,-1.,2.60927675461843E-32));
#24032=DIRECTION('ref_axis',(0.560568426943322,0.,-0.828108108108047));
#24033=DIRECTION('center_axis',(6.02124417213198E-17,-1.,2.60927675461843E-32));
#24034=DIRECTION('ref_axis',(0.560568426943322,0.,-0.828108108108047));
#24035=DIRECTION('center_axis',(-1.,0.,-8.67628499512335E-13));
#24036=DIRECTION('ref_axis',(8.67628499512335E-13,-5.79319727271681E-31,
-1.));
#24037=DIRECTION('',(8.67628499512335E-13,5.22159376950964E-29,-1.));
#24038=DIRECTION('',(0.,-1.,0.));
#24039=DIRECTION('',(-6.13505995555881E-13,-0.707106781186547,0.707106781186548));
#24040=DIRECTION('',(5.67373952042745E-44,-1.,-6.53936508957056E-32));
#24041=DIRECTION('center_axis',(-1.,0.,-8.67628499512335E-13));
#24042=DIRECTION('ref_axis',(8.67628499512335E-13,-5.79319727271681E-31,
-1.));
#24043=DIRECTION('',(8.67628499512335E-13,5.22159376950964E-29,-1.));
#24044=DIRECTION('',(-5.67373952042745E-44,1.,6.53936508957056E-32));
#24045=DIRECTION('',(-6.13505995555881E-13,0.707106781186547,0.707106781186548));
#24046=DIRECTION('',(0.,1.,0.));
#24047=DIRECTION('center_axis',(-4.64905891561784E-16,0.,-1.));
#24048=DIRECTION('ref_axis',(1.,2.80259692864963E-45,-4.64905891561784E-16));
#24049=DIRECTION('',(1.,6.02124417213198E-17,-4.64905891561784E-16));
#24050=DIRECTION('',(-1.,1.92408737950894E-15,4.64905891561784E-16));
#24051=DIRECTION('',(-0.707106781186548,-0.707106781186547,3.28738108536916E-16));
#24052=DIRECTION('',(6.02124417213198E-17,-1.,-2.79931189015622E-32));
#24053=DIRECTION('center_axis',(-1.,0.,-8.67628499512335E-13));
#24054=DIRECTION('ref_axis',(8.67628499512335E-13,-5.79319727271681E-31,
-1.));
#24055=DIRECTION('',(-8.67628499512335E-13,-4.96193574268823E-11,1.));
#24056=DIRECTION('',(4.61918851910391E-44,-1.,-5.32392437742675E-32));
#24057=DIRECTION('',(8.67628499512335E-13,5.22159376950964E-29,-1.));
#24058=DIRECTION('',(0.,-1.,0.));
#24059=DIRECTION('center_axis',(0.,-1.,0.));
#24060=DIRECTION('ref_axis',(1.,0.,-5.00979119302536E-12));
#24061=DIRECTION('center_axis',(0.700909264299845,-0.713250449154187,1.06495728142558E-15));
#24062=DIRECTION('ref_axis',(0.713250449154187,0.700909264299845,-3.57323581859403E-12));
#24063=DIRECTION('center_axis',(0.999847695156391,-0.0174524064372835,1.51916251861363E-15));
#24064=DIRECTION('ref_axis',(0.0174524064372835,0.999847695156391,-8.74329120666019E-14));
#24065=DIRECTION('center_axis',(-6.02124417213198E-17,1.,-2.60927675461843E-32));
#24066=DIRECTION('ref_axis',(1.,0.,-5.00979119302536E-12));
#24067=DIRECTION('',(0.,-1.,0.));
#24068=DIRECTION('center_axis',(0.,-1.,0.));
#24069=DIRECTION('ref_axis',(0.828108108108418,0.,0.560568426942775));
#24070=DIRECTION('center_axis',(-1.02201073032319E-15,-0.713250449154181,
0.700909264299851));
#24071=DIRECTION('ref_axis',(-1.07158130997516E-15,0.700909264299851,0.713250449154181));
#24072=DIRECTION('center_axis',(6.02124417213198E-17,-1.,2.60927675461843E-32));
#24073=DIRECTION('ref_axis',(0.828108108108418,0.,0.560568426942775));
#24074=DIRECTION('center_axis',(6.02124417213198E-17,-1.,2.60927675461843E-32));
#24075=DIRECTION('ref_axis',(0.828108108108418,0.,0.560568426942775));
#24076=DIRECTION('center_axis',(0.700909264299845,-0.713250449154187,1.06495728142558E-15));
#24077=DIRECTION('ref_axis',(0.713250449154187,0.700909264299845,1.19764969938401E-15));
#24078=DIRECTION('center_axis',(-6.02124417213198E-17,1.,-2.60927675461843E-32));
#24079=DIRECTION('ref_axis',(0.828108108108418,0.,0.560568426942775));
#24080=DIRECTION('',(0.,-1.,0.));
#24081=DIRECTION('center_axis',(0.,-1.,0.));
#24082=DIRECTION('ref_axis',(0.560568426942125,0.,0.828108108108858));
#24083=DIRECTION('center_axis',(-1.51811166660813E-15,-0.0174524064372836,
0.999847695156391));
#24084=DIRECTION('ref_axis',(-2.664208725992E-17,0.999847695156391,0.0174524064372836));
#24085=DIRECTION('center_axis',(-1.02201073032319E-15,-0.713250449154181,
0.700909264299851));
#24086=DIRECTION('ref_axis',(-9.89833838717548E-16,0.700909264299851,0.713250449154181));
#24087=DIRECTION('center_axis',(-6.02124417213198E-17,1.,-2.60927675461843E-32));
#24088=DIRECTION('ref_axis',(0.560568426942125,0.,0.828108108108858));
#24089=DIRECTION('center_axis',(0.,-1.,0.));
#24090=DIRECTION('ref_axis',(0.828108108108829,0.,-0.560568426942167));
#24091=DIRECTION('center_axis',(-6.02124417213198E-17,1.,-2.60927675461843E-32));
#24092=DIRECTION('ref_axis',(0.828108108108829,0.,-0.560568426942167));
#24093=DIRECTION('',(0.,-1.,0.));
#24094=DIRECTION('center_axis',(0.999847695156391,-0.0174524064372835,1.51916251861363E-15));
#24095=DIRECTION('ref_axis',(0.0174524064372835,0.999847695156391,2.42200793274045E-17));
#24096=DIRECTION('center_axis',(0.700909264299845,-0.713250449154187,1.06495728142558E-15));
#24097=DIRECTION('ref_axis',(0.713250449154187,0.700909264299845,1.1878006064711E-15));
#24098=DIRECTION('center_axis',(-1.,0.,-8.67628499512335E-13));
#24099=DIRECTION('ref_axis',(8.67628499512335E-13,-5.79319727271681E-31,
-1.));
#24100=DIRECTION('',(8.67628499512335E-13,5.22159376950964E-29,-1.));
#24101=DIRECTION('',(-2.1384182212495E-44,1.,2.46467033119755E-32));
#24102=DIRECTION('',(-8.67628499512335E-13,-4.96193574268823E-11,1.));
#24103=DIRECTION('center_axis',(4.64905891561784E-16,0.,1.));
#24104=DIRECTION('ref_axis',(-1.,-2.80259692864963E-45,4.64905891561784E-16));
#24105=DIRECTION('',(-1.,-6.02124417213198E-17,4.64905891561784E-16));
#24106=DIRECTION('',(-6.02124417213198E-17,1.,2.79931189015621E-32));
#24107=DIRECTION('',(0.707106781186546,0.70710678118655,-3.28738108536915E-16));
#24108=DIRECTION('',(1.,2.04451226295158E-15,-4.64905891561784E-16));
#24109=DIRECTION('center_axis',(-1.51811166660813E-15,-0.0174524064372836,
0.999847695156391));
#24110=DIRECTION('ref_axis',(-1.,-6.02124417213198E-17,-1.51939392966847E-15));
#24111=DIRECTION('',(-1.,-6.02124417213198E-17,-1.51939392966847E-15));
#24112=DIRECTION('center_axis',(6.02124417213198E-17,-1.,2.60927675461843E-32));
#24113=DIRECTION('ref_axis',(-1.,-6.02124417213198E-17,-1.51939392966847E-15));
#24114=DIRECTION('center_axis',(-6.02124417213198E-17,1.,-2.60927675461843E-32));
#24115=DIRECTION('ref_axis',(-1.,-6.02124417213198E-17,-1.51939392966847E-15));
#24116=DIRECTION('',(0.707106781186546,-0.707106781186548,1.1609693565858E-15));
#24117=DIRECTION('center_axis',(6.02124417213198E-17,-1.,2.60927675461843E-32));
#24118=DIRECTION('ref_axis',(-1.,-6.02124417213198E-17,-1.51939392966847E-15));
#24119=DIRECTION('center_axis',(6.02124417213198E-17,-1.,2.60927675461843E-32));
#24120=DIRECTION('ref_axis',(-1.,-6.02124417213198E-17,-1.51939392966847E-15));
#24121=DIRECTION('center_axis',(-6.02124417213198E-17,1.,-2.60927675461843E-32));
#24122=DIRECTION('ref_axis',(-1.,-6.02124417213198E-17,-1.51939392966847E-15));
#24123=DIRECTION('center_axis',(-0.999847695156391,-0.0174524064372837,
-1.51916251861363E-15));
#24124=DIRECTION('ref_axis',(1.51939392966847E-15,3.89938443409397E-32,
-1.));
#24125=DIRECTION('',(1.51939392966847E-15,6.53936508957056E-32,-1.));
#24126=DIRECTION('center_axis',(-0.700909264299851,-0.713250449154181,-1.06495728142559E-15));
#24127=DIRECTION('ref_axis',(1.51939392966847E-15,2.11007687440828E-30,
-1.));
#24128=DIRECTION('',(-1.51939392966847E-15,-6.53936508957056E-32,1.));
#24129=DIRECTION('center_axis',(6.02124417213198E-17,-1.,2.60927675461843E-32));
#24130=DIRECTION('ref_axis',(-1.,-6.02124417213198E-17,-1.51939392966847E-15));
#24131=DIRECTION('center_axis',(-6.02124417213198E-17,1.,-2.60927675461843E-32));
#24132=DIRECTION('ref_axis',(-1.,-6.02124417213198E-17,-1.51939392966847E-15));
#24133=DIRECTION('',(0.707106781186546,-0.707106781186548,1.1609693565858E-15));
#24134=DIRECTION('center_axis',(6.02124417213198E-17,-1.,2.60927675461843E-32));
#24135=DIRECTION('ref_axis',(-1.,-6.02124417213198E-17,-1.51939392966847E-15));
#24136=DIRECTION('center_axis',(6.02124417213198E-17,-1.,2.60927675461843E-32));
#24137=DIRECTION('ref_axis',(-1.,-6.02124417213198E-17,-1.51939392966847E-15));
#24138=DIRECTION('center_axis',(-6.02124417213198E-17,1.,-2.60927675461843E-32));
#24139=DIRECTION('ref_axis',(-1.,-6.02124417213198E-17,-1.51939392966847E-15));
#24140=DIRECTION('center_axis',(1.52021337061914E-15,-0.0174524064372836,
-0.999847695156391));
#24141=DIRECTION('ref_axis',(1.,6.02124417213199E-17,1.51939392966848E-15));
#24142=DIRECTION('',(1.,6.02124417213198E-17,1.51939392966847E-15));
#24143=DIRECTION('center_axis',(1.10790383252799E-15,-0.713250449154181,
-0.700909264299851));
#24144=DIRECTION('ref_axis',(1.,6.02124417213211E-17,1.51939392966847E-15));
#24145=DIRECTION('',(-1.,-6.02124417213198E-17,-1.51939392966847E-15));
#24146=DIRECTION('center_axis',(6.02124417213198E-17,-1.,2.60927675461843E-32));
#24147=DIRECTION('ref_axis',(-1.,-6.02124417213198E-17,-1.51939392966847E-15));
#24148=DIRECTION('center_axis',(-6.02124417213198E-17,1.,-2.60927675461843E-32));
#24149=DIRECTION('ref_axis',(-1.,-6.02124417213198E-17,-1.51939392966847E-15));
#24150=DIRECTION('',(0.707106781186546,-0.707106781186548,1.1609693565858E-15));
#24151=DIRECTION('center_axis',(6.02124417213198E-17,-1.,2.60927675461843E-32));
#24152=DIRECTION('ref_axis',(-1.,-6.02124417213198E-17,-1.51939392966847E-15));
#24153=DIRECTION('center_axis',(6.02124417213198E-17,-1.,2.60927675461843E-32));
#24154=DIRECTION('ref_axis',(-1.,-6.02124417213198E-17,-1.51939392966847E-15));
#24155=DIRECTION('center_axis',(-6.02124417213198E-17,1.,-2.60927675461843E-32));
#24156=DIRECTION('ref_axis',(-1.,-6.02124417213198E-17,-1.51939392966847E-15));
#24157=DIRECTION('center_axis',(0.700909264299845,-0.713250449154187,1.06495728142558E-15));
#24158=DIRECTION('ref_axis',(-1.51939392966847E-15,1.65690546530681E-30,
1.));
#24159=DIRECTION('',(1.51939392966847E-15,6.53936508957056E-32,-1.));
#24160=DIRECTION('',(0.584067929597373,0.573961955888994,-0.573961955888993));
#24161=DIRECTION('',(1.51939392966847E-15,6.53936508957056E-32,-1.));
#24162=DIRECTION('center_axis',(1.51939392966847E-15,6.53936508957056E-32,
-1.));
#24163=DIRECTION('ref_axis',(1.,6.02124417213198E-17,1.51939392966847E-15));
#24164=DIRECTION('',(1.,6.02124417213198E-17,1.51939392966847E-15));
#24165=DIRECTION('',(-0.0174524064382658,-0.999847695156374,-2.6517080400408E-17));
#24166=DIRECTION('',(1.,6.02124417213198E-17,1.51939392966847E-15));
#24167=DIRECTION('center_axis',(1.1169503768152E-15,-0.707106781186548,
-0.707106781186547));
#24168=DIRECTION('ref_axis',(1.,6.02124417213228E-17,1.51939392966847E-15));
#24169=DIRECTION('',(1.01152894254293E-12,-0.707106781186547,0.707106781186548));
#24170=DIRECTION('',(-1.,-6.02124417213198E-17,-1.51939392966847E-15));
#24171=DIRECTION('',(0.0123416547519202,0.707052927141238,-0.707052927141238));
#24172=DIRECTION('center_axis',(0.707106781186547,4.2576625852945E-17,0.707106781186549));
#24173=DIRECTION('ref_axis',(-6.02124417213198E-17,1.,-9.64348767934759E-33));
#24174=DIRECTION('',(0.707106781186548,4.25766258529451E-17,-0.707106781186547));
#24175=DIRECTION('',(-6.02124417213198E-17,1.,-2.60927675461843E-32));
#24176=DIRECTION('',(-0.707106781186548,-4.25766258529451E-17,0.707106781186547));
#24177=DIRECTION('center_axis',(6.02124417213198E-17,-1.,2.60927675461843E-32));
#24178=DIRECTION('ref_axis',(1.,6.02124417213198E-17,1.51939392966847E-15));
#24179=DIRECTION('',(1.,6.02124417213198E-17,1.51939392966847E-15));
#24180=DIRECTION('',(1.00179694968482E-12,6.02945476819473E-29,-1.));
#24181=DIRECTION('',(1.,6.02124417213198E-17,1.51939392966847E-15));
#24182=DIRECTION('',(1.51939392966847E-15,6.53936508957056E-32,-1.));
#24183=DIRECTION('center_axis',(6.02124417213198E-17,-1.,2.60927675461843E-32));
#24184=DIRECTION('ref_axis',(-1.,-6.02124417213198E-17,-1.51939392966847E-15));
#24185=DIRECTION('center_axis',(6.02124417213198E-17,-1.,2.60927675461843E-32));
#24186=DIRECTION('ref_axis',(-1.,-6.02124417213198E-17,-1.51939392966847E-15));
#24187=DIRECTION('center_axis',(-6.02124417213198E-17,1.,-2.60927675461843E-32));
#24188=DIRECTION('ref_axis',(1.,6.02124417213198E-17,1.51939392966847E-15));
#24189=DIRECTION('center_axis',(6.02124417213198E-17,-1.,2.60927675461843E-32));
#24190=DIRECTION('ref_axis',(1.,6.02124417213198E-17,1.51939392966847E-15));
#24191=DIRECTION('center_axis',(6.02124417213198E-17,-1.,2.60927675461843E-32));
#24192=DIRECTION('ref_axis',(1.,6.02124417213198E-17,1.51939392966847E-15));
#24193=DIRECTION('',(6.02124417213198E-17,-1.,2.60927675461843E-32));
#24194=DIRECTION('center_axis',(6.02124417213198E-17,-1.,2.60927675461843E-32));
#24195=DIRECTION('ref_axis',(1.,6.02124417213198E-17,1.51939392966847E-15));
#24196=DIRECTION('center_axis',(6.02124417213198E-17,-1.,2.60927675461843E-32));
#24197=DIRECTION('ref_axis',(1.,6.02124417213198E-17,1.51939392966847E-15));
#24198=DIRECTION('',(6.02124417213198E-17,-1.,2.60927675461843E-32));
#24199=DIRECTION('center_axis',(6.02124417213198E-17,-1.,2.60927675461843E-32));
#24200=DIRECTION('ref_axis',(-1.,-6.02124417213198E-17,-1.51939392966847E-15));
#24201=DIRECTION('center_axis',(-6.02124417213198E-17,1.,-2.60927675461843E-32));
#24202=DIRECTION('ref_axis',(-1.,-6.02124417213198E-17,-1.51939392966847E-15));
#24203=DIRECTION('',(0.707106781186546,-0.707106781186548,1.1609693565858E-15));
#24204=DIRECTION('center_axis',(-6.02124417213198E-17,1.,-2.60927675461843E-32));
#24205=DIRECTION('ref_axis',(-1.,-6.02124417213198E-17,-1.51939392966847E-15));
#24206=DIRECTION('center_axis',(6.02124417213198E-17,-1.,2.60927675461843E-32));
#24207=DIRECTION('ref_axis',(1.,6.02124417213198E-17,1.51939392966847E-15));
#24208=DIRECTION('center_axis',(6.02124417213198E-17,-1.,2.60927675461843E-32));
#24209=DIRECTION('ref_axis',(1.,6.02124417213198E-17,1.51939392966847E-15));
#24210=DIRECTION('',(6.02124417213198E-17,-1.,2.60927675461843E-32));
#24211=DIRECTION('center_axis',(6.02124417213198E-17,-1.,2.60927675461843E-32));
#24212=DIRECTION('ref_axis',(1.,6.02124417213198E-17,1.51939392966847E-15));
#24213=DIRECTION('center_axis',(6.02124417213198E-17,-1.,2.60927675461843E-32));
#24214=DIRECTION('ref_axis',(1.,6.02124417213198E-17,1.51939392966847E-15));
#24215=DIRECTION('',(6.02124417213198E-17,-1.,2.60927675461843E-32));
#24216=DIRECTION('center_axis',(6.02124417213198E-17,-1.,2.60927675461843E-32));
#24217=DIRECTION('ref_axis',(-0.707106781186546,-4.2576625852945E-17,-0.707106781186549));
#24218=DIRECTION('center_axis',(6.02124417213198E-17,-1.,2.60927675461843E-32));
#24219=DIRECTION('ref_axis',(-0.707106781186546,-4.2576625852945E-17,-0.707106781186549));
#24220=DIRECTION('',(6.02124417213198E-17,-1.,2.60927675461843E-32));
#24221=DIRECTION('center_axis',(-6.02124417213198E-17,1.,-2.60927675461843E-32));
#24222=DIRECTION('ref_axis',(-0.707106781186546,-4.2576625852945E-17,-0.707106781186549));
#24223=DIRECTION('',(-6.02124417213198E-17,1.,-2.60927675461843E-32));
#24224=DIRECTION('center_axis',(-1.31753519791844E-15,-5.32392437742675E-32,
1.));
#24225=DIRECTION('ref_axis',(-6.02124417213198E-17,1.,-2.60927675461841E-32));
#24226=DIRECTION('',(0.0174524064382658,0.999847695156374,2.6517080400408E-17));
#24227=DIRECTION('',(-1.,-6.02124417213198E-17,9.98682464801081E-13));
#24228=DIRECTION('',(-1.,-6.02124417213198E-17,9.98682464801081E-13));
#24229=DIRECTION('center_axis',(6.02124417213198E-17,-1.,2.60927675461843E-32));
#24230=DIRECTION('ref_axis',(1.,6.02124417213198E-17,1.51939392966847E-15));
#24231=DIRECTION('',(-0.707106781186549,-4.25766258529451E-17,0.707106781186546));
#24232=DIRECTION('',(-1.,-6.02124417213198E-17,-1.00165684600473E-12));
#24233=DIRECTION('',(-0.707106781186546,-4.25766258529449E-17,-0.707106781186549));
#24234=DIRECTION('',(1.00165684600473E-12,6.02861116972749E-29,-1.));
#24235=DIRECTION('',(0.707106781186548,4.25766258529451E-17,-0.707106781186547));
#24236=DIRECTION('',(1.,6.02124417213198E-17,1.51939392966847E-15));
#24237=DIRECTION('',(0.707106781186547,4.2576625852945E-17,0.707106781186548));
#24238=DIRECTION('center_axis',(6.02124417213198E-17,-1.,2.60927675461843E-32));
#24239=DIRECTION('ref_axis',(-1.51939392966847E-15,-6.53936508957055E-32,
1.));
#24240=DIRECTION('',(1.,6.02124417213198E-17,-9.98682464801081E-13));
#24241=DIRECTION('center_axis',(6.02124417213198E-17,-1.,2.60927675461843E-32));
#24242=DIRECTION('ref_axis',(1.,6.02124417213198E-17,1.51939392966847E-15));
#24243=DIRECTION('center_axis',(6.02124417213198E-17,-1.,2.60927675461843E-32));
#24244=DIRECTION('ref_axis',(1.,6.02124417213198E-17,1.51939392966847E-15));
#24245=DIRECTION('center_axis',(6.02124417213198E-17,-1.,2.60927675461843E-32));
#24246=DIRECTION('ref_axis',(1.,6.02124417213198E-17,1.51939392966847E-15));
#24247=DIRECTION('center_axis',(6.02124417213198E-17,-1.,2.60927675461843E-32));
#24248=DIRECTION('ref_axis',(1.,6.02124417213198E-17,1.51939392966847E-15));
#24249=DIRECTION('center_axis',(6.02124417213198E-17,-1.,2.60927675461843E-32));
#24250=DIRECTION('ref_axis',(-1.51939392966847E-15,-6.53936508957055E-32,
1.));
#24251=DIRECTION('',(6.02124417213198E-17,-1.,2.60927675461843E-32));
#24252=DIRECTION('center_axis',(-6.02124417213198E-17,1.,-2.60927675461843E-32));
#24253=DIRECTION('ref_axis',(-1.51939392966847E-15,-6.53936508957055E-32,
1.));
#24254=DIRECTION('',(-6.02124417213198E-17,1.,-2.60927675461843E-32));
#24255=DIRECTION('center_axis',(0.707106781186549,4.25766258529451E-17,
-0.707106781186547));
#24256=DIRECTION('ref_axis',(-6.02124417213198E-17,1.,-2.60096122749369E-32));
#24257=DIRECTION('',(6.02124417213198E-17,-1.,2.60927675461843E-32));
#24258=DIRECTION('',(0.707106781186547,4.2576625852945E-17,0.707106781186548));
#24259=DIRECTION('',(-6.02124417213198E-17,1.,-2.60927675461843E-32));
#24260=DIRECTION('',(0.707106781186547,4.2576625852945E-17,0.707106781186548));
#24261=DIRECTION('',(6.02124417213198E-17,-1.,2.60927675461843E-32));
#24262=DIRECTION('',(0.707106781186547,4.2576625852945E-17,0.707106781186548));
#24263=DIRECTION('center_axis',(1.51939392966847E-15,2.46467033119755E-32,
-1.));
#24264=DIRECTION('ref_axis',(1.,-1.41646290028709E-16,1.51939392966847E-15));
#24265=DIRECTION('',(1.,6.02124417213198E-17,-9.98682464801081E-13));
#24266=DIRECTION('',(-0.0174524064382658,-0.999847695156374,-2.6517080400408E-17));
#24267=DIRECTION('center_axis',(0.577350269189625,-0.577350269189626,0.577350269189627));
#24268=DIRECTION('ref_axis',(-1.15783932620466E-15,0.707106781186548,0.707106781186548));
#24269=DIRECTION('',(-1.1169503768152E-15,0.707106781186547,0.707106781186548));
#24270=DIRECTION('',(-0.707106781186546,-0.707106781186549,-1.00421455866691E-12));
#24271=DIRECTION('center_axis',(0.577350269189625,-0.577350269189622,-0.577350269189631));
#24272=DIRECTION('ref_axis',(0.707106781186546,0.707106781186549,9.40034155039792E-16));
#24273=DIRECTION('',(-0.707106781186551,-4.25766258529452E-17,-0.707106781186544));
#24274=DIRECTION('',(0.707106781186546,0.707106781186549,1.07437375096225E-15));
#24275=DIRECTION('center_axis',(0.707106781186544,4.25766258529448E-17,
-0.707106781186551));
#24276=DIRECTION('ref_axis',(-6.02124417213198E-17,1.,-2.25152429480529E-32));
#24277=DIRECTION('',(0.707106781186551,4.25766258529452E-17,0.707106781186544));
#24278=DIRECTION('',(6.02124417213198E-17,-1.,2.60927675461843E-32));
#24279=DIRECTION('center_axis',(0.707106781186549,-0.707106781186546,1.27063530829773E-15));
#24280=DIRECTION('ref_axis',(-1.51939392966847E-15,2.77555756156293E-16,
1.));
#24281=DIRECTION('',(-1.00179694968482E-12,-6.02945476819473E-29,1.));
#24282=DIRECTION('center_axis',(-1.03179712510931E-15,-0.707106781186548,
0.707106781186547));
#24283=DIRECTION('ref_axis',(-1.,-6.02124417213168E-17,-1.51939392966847E-15));
#24284=DIRECTION('',(-1.,-6.02124417213198E-17,-1.51939392966847E-15));
#24285=DIRECTION('',(0.0123416547519181,0.707052927141238,0.707052927141238));
#24286=DIRECTION('',(0.584067929597371,0.573961955888994,0.573961955888995));
#24287=DIRECTION('center_axis',(6.02124417213198E-17,-1.,2.60927675461843E-32));
#24288=DIRECTION('ref_axis',(-0.707106781186548,-4.25766258529451E-17,-0.707106781186547));
#24289=DIRECTION('center_axis',(-6.02124417213198E-17,1.,-2.60927675461843E-32));
#24290=DIRECTION('ref_axis',(-0.707106781186548,-4.25766258529451E-17,-0.707106781186547));
#24291=DIRECTION('',(-6.02124417213198E-17,1.,-2.60927675461843E-32));
#24292=DIRECTION('center_axis',(-6.02124417213198E-17,1.,-2.60927675461843E-32));
#24293=DIRECTION('ref_axis',(-0.707106781186548,-4.25766258529451E-17,-0.707106781186547));
#24294=DIRECTION('',(6.02124417213198E-17,-1.,2.60927675461843E-32));
#24295=DIRECTION('center_axis',(1.51939392966847E-15,6.53936508957056E-32,
-1.));
#24296=DIRECTION('ref_axis',(1.,6.02124417213198E-17,1.51939392966847E-15));
#24297=DIRECTION('',(1.,6.02124417213198E-17,1.51939392966847E-15));
#24298=DIRECTION('',(6.02124417213198E-17,-1.,2.60927675461843E-32));
#24299=DIRECTION('',(1.,6.02124417213198E-17,1.51939392966847E-15));
#24300=DIRECTION('center_axis',(6.02124417213198E-17,-1.,2.60927675461843E-32));
#24301=DIRECTION('ref_axis',(0.707106781186547,4.2576625852945E-17,-0.707106781186548));
#24302=DIRECTION('center_axis',(-6.02124417213198E-17,1.,-2.60927675461843E-32));
#24303=DIRECTION('ref_axis',(0.707106781186547,4.2576625852945E-17,-0.707106781186548));
#24304=DIRECTION('',(-6.02124417213198E-17,1.,-2.60927675461843E-32));
#24305=DIRECTION('center_axis',(-6.02124417213198E-17,1.,-2.60927675461843E-32));
#24306=DIRECTION('ref_axis',(0.707106781186547,4.2576625852945E-17,-0.707106781186548));
#24307=DIRECTION('center_axis',(1.,6.02124417213198E-17,1.51939392966847E-15));
#24308=DIRECTION('ref_axis',(6.02124417213198E-17,-1.,2.60927675461843E-32));
#24309=DIRECTION('',(-1.51939392966847E-15,-6.53936508957056E-32,1.));
#24310=DIRECTION('',(6.02124417213198E-17,-1.,2.60927675461843E-32));
#24311=DIRECTION('',(-1.51939392966847E-15,-6.53936508957056E-32,1.));
#24312=DIRECTION('center_axis',(6.02124417213198E-17,-1.,2.60927675461843E-32));
#24313=DIRECTION('ref_axis',(0.707106781186545,4.25766258529449E-17,0.70710678118655));
#24314=DIRECTION('center_axis',(-6.02124417213198E-17,1.,-2.60927675461843E-32));
#24315=DIRECTION('ref_axis',(0.707106781186545,4.25766258529449E-17,0.70710678118655));
#24316=DIRECTION('',(-6.02124417213198E-17,1.,-2.60927675461843E-32));
#24317=DIRECTION('center_axis',(-6.02124417213198E-17,1.,-2.60927675461843E-32));
#24318=DIRECTION('ref_axis',(0.707106781186545,4.25766258529449E-17,0.70710678118655));
#24319=DIRECTION('center_axis',(-1.51939392966847E-15,-6.53936508957056E-32,
1.));
#24320=DIRECTION('ref_axis',(-6.02124417213198E-17,1.,-2.60927675461842E-32));
#24321=DIRECTION('',(-1.,-6.02124417213198E-17,-1.51939392966847E-15));
#24322=DIRECTION('',(6.02124417213198E-17,-1.,2.60927675461843E-32));
#24323=DIRECTION('',(-1.,-6.02124417213198E-17,-1.51939392966847E-15));
#24324=DIRECTION('center_axis',(6.02124417213198E-17,-1.,2.60927675461843E-32));
#24325=DIRECTION('ref_axis',(-0.707106781186547,-4.2576625852945E-17,0.707106781186548));
#24326=DIRECTION('center_axis',(-6.02124417213198E-17,1.,-2.60927675461843E-32));
#24327=DIRECTION('ref_axis',(-0.707106781186547,-4.2576625852945E-17,0.707106781186548));
#24328=DIRECTION('',(-6.02124417213198E-17,1.,-2.60927675461843E-32));
#24329=DIRECTION('center_axis',(-6.02124417213198E-17,1.,-2.60927675461843E-32));
#24330=DIRECTION('ref_axis',(-0.707106781186547,-4.2576625852945E-17,0.707106781186548));
#24331=DIRECTION('center_axis',(6.02124417213198E-17,-1.,2.60927675461843E-32));
#24332=DIRECTION('ref_axis',(1.,6.02124417213198E-17,1.51939392966847E-15));
#24333=DIRECTION('',(1.51939392966847E-15,6.53936508957056E-32,-1.));
#24334=DIRECTION('center_axis',(-1.,-6.02124417213198E-17,-1.51939392966847E-15));
#24335=DIRECTION('ref_axis',(1.51939392966847E-15,6.53936508957056E-32,
-1.));
#24336=DIRECTION('',(1.51939392966847E-15,6.53936508957056E-32,-1.));
#24337=DIRECTION('center_axis',(0.999847695156391,-0.0174524064372835,1.51916251861363E-15));
#24338=DIRECTION('ref_axis',(-1.51939392966847E-15,-9.04549301518072E-32,
1.));
#24339=DIRECTION('center_axis',(0.700909264299845,-0.713250449154187,1.06495728142558E-15));
#24340=DIRECTION('ref_axis',(-1.51939392966847E-15,1.65690546530681E-30,
1.));
#24341=DIRECTION('',(-1.51939392966847E-15,-6.53936508957056E-32,1.));
#24342=DIRECTION('center_axis',(6.02124417213198E-17,-1.,2.60927675461843E-32));
#24343=DIRECTION('ref_axis',(1.,6.02124417213198E-17,1.51939392966847E-15));
#24344=DIRECTION('center_axis',(6.02124417213198E-17,-1.,2.60927675461843E-32));
#24345=DIRECTION('ref_axis',(1.,6.02124417213198E-17,1.51939392966847E-15));
#24346=DIRECTION('',(6.02124417213198E-17,-1.,2.60927675461843E-32));
#24347=DIRECTION('center_axis',(-1.51939392966847E-15,-6.53936508957056E-32,
1.));
#24348=DIRECTION('ref_axis',(-6.02124417213198E-17,1.,-2.60927675461842E-32));
#24349=DIRECTION('',(-1.,-6.02124417213198E-17,-1.51939392966847E-15));
#24350=DIRECTION('',(0.0174524064382658,0.999847695156374,2.6517080400408E-17));
#24351=DIRECTION('center_axis',(1.,6.02124417213198E-17,1.79694968582476E-15));
#24352=DIRECTION('ref_axis',(6.02124417213198E-17,-1.,2.60927675461843E-32));
#24353=DIRECTION('',(-1.00179694968482E-12,-6.02945476819473E-29,1.));
#24354=DIRECTION('center_axis',(-6.02124417213198E-17,1.,-2.60927675461843E-32));
#24355=DIRECTION('ref_axis',(0.0161939654040152,9.75078198126308E-19,-0.999868869144596));
#24356=DIRECTION('center_axis',(6.02124417213198E-17,-1.,2.60927675461843E-32));
#24357=DIRECTION('ref_axis',(0.0161939654068418,9.75078198296505E-19,-0.99986886914455));
#24358=DIRECTION('',(6.02124417213198E-17,-1.,2.60927675461843E-32));
#24359=DIRECTION('center_axis',(-6.02124417213198E-17,1.,-2.60927675461843E-32));
#24360=DIRECTION('ref_axis',(0.0161939654068418,9.75078198296505E-19,-0.99986886914455));
#24361=DIRECTION('',(-6.02124417213198E-17,1.,-2.60927675461843E-32));
#24362=DIRECTION('center_axis',(-6.02124417213198E-17,1.,-2.60927675461843E-32));
#24363=DIRECTION('ref_axis',(-1.51939392966847E-15,-6.53936508957055E-32,
1.));
#24364=DIRECTION('',(-0.707106781186549,-4.25766258529451E-17,0.707106781186546));
#24365=DIRECTION('center_axis',(-6.02124417213198E-17,1.,-2.60927675461843E-32));
#24366=DIRECTION('ref_axis',(-0.999868869144596,-6.02045460123309E-17,-0.0161939654040152));
#24367=DIRECTION('center_axis',(6.02124417213198E-17,-1.,2.60927675461843E-32));
#24368=DIRECTION('ref_axis',(-0.99986886914455,-6.02045460123282E-17,-0.0161939654068418));
#24369=DIRECTION('center_axis',(-6.02124417213198E-17,1.,-2.60927675461843E-32));
#24370=DIRECTION('ref_axis',(-0.99986886914455,-6.02045460123282E-17,-0.0161939654068418));
#24371=DIRECTION('center_axis',(-6.02124417213198E-17,1.,-2.60927675461843E-32));
#24372=DIRECTION('ref_axis',(-1.51939392966847E-15,-6.53936508957055E-32,
1.));
#24373=DIRECTION('center_axis',(-6.02124417213198E-17,1.,-2.60927675461843E-32));
#24374=DIRECTION('ref_axis',(-0.0161939654040153,-9.75078198126314E-19,
0.999868869144596));
#24375=DIRECTION('center_axis',(6.02124417213198E-17,-1.,2.60927675461843E-32));
#24376=DIRECTION('ref_axis',(-0.0161939654068419,-9.75078198296511E-19,
0.99986886914455));
#24377=DIRECTION('',(6.02124417213198E-17,-1.,2.60927675461843E-32));
#24378=DIRECTION('center_axis',(-6.02124417213198E-17,1.,-2.60927675461843E-32));
#24379=DIRECTION('ref_axis',(-0.0161939654068419,-9.75078198296511E-19,
0.99986886914455));
#24380=DIRECTION('',(-6.02124417213198E-17,1.,-2.60927675461843E-32));
#24381=DIRECTION('center_axis',(-6.02124417213198E-17,1.,-2.60927675461843E-32));
#24382=DIRECTION('ref_axis',(-1.51939392966847E-15,-6.53936508957055E-32,
1.));
#24383=DIRECTION('',(0.707106781186548,4.25766258529451E-17,-0.707106781186547));
#24384=DIRECTION('center_axis',(0.707106781186546,4.25766258529449E-17,
0.707106781186549));
#24385=DIRECTION('ref_axis',(-6.02124417213198E-17,1.,1.32224183220761E-32));
#24386=DIRECTION('',(-0.707106781186549,-4.25766258529451E-17,0.707106781186546));
#24387=DIRECTION('',(-0.707106781186549,-4.25766258529451E-17,0.707106781186546));
#24388=DIRECTION('',(6.02124417213198E-17,-1.,2.60927675461843E-32));
#24389=DIRECTION('center_axis',(-0.707106781186547,-4.2576625852945E-17,
-0.707106781186549));
#24390=DIRECTION('ref_axis',(6.02124417213198E-17,-1.,9.64348767934759E-33));
#24391=DIRECTION('',(0.707106781186548,4.25766258529451E-17,-0.707106781186547));
#24392=DIRECTION('',(6.02124417213198E-17,-1.,2.60927675461843E-32));
#24393=DIRECTION('',(6.02124417213198E-17,-1.,2.60927675461843E-32));
#24394=DIRECTION('',(0.707106781186548,4.25766258529451E-17,-0.707106781186547));
#24395=DIRECTION('center_axis',(-6.02124417213198E-17,1.,-2.60927675461843E-32));
#24396=DIRECTION('ref_axis',(0.999868869144596,6.02045460123309E-17,0.0161939654040153));
#24397=DIRECTION('center_axis',(6.02124417213198E-17,-1.,2.60927675461843E-32));
#24398=DIRECTION('ref_axis',(0.99986886914455,6.02045460123282E-17,0.0161939654068419));
#24399=DIRECTION('',(6.02124417213198E-17,-1.,2.60927675461843E-32));
#24400=DIRECTION('center_axis',(-6.02124417213198E-17,1.,-2.60927675461843E-32));
#24401=DIRECTION('ref_axis',(0.99986886914455,6.02045460123282E-17,0.0161939654068419));
#24402=DIRECTION('',(-6.02124417213198E-17,1.,-2.60927675461843E-32));
#24403=DIRECTION('center_axis',(-6.02124417213198E-17,1.,-2.60927675461843E-32));
#24404=DIRECTION('ref_axis',(-1.51939392966847E-15,-6.53936508957055E-32,
1.));
#24405=DIRECTION('',(-0.707106781186546,-4.25766258529449E-17,-0.707106781186549));
#24406=DIRECTION('center_axis',(-0.707106781186549,-4.25766258529451E-17,
0.707106781186546));
#24407=DIRECTION('ref_axis',(-0.707106781186546,-4.25766258529449E-17,-0.707106781186549));
#24408=DIRECTION('',(-0.707106781186546,-4.25766258529449E-17,-0.707106781186549));
#24409=DIRECTION('',(6.02124417213198E-17,-1.,2.60927675461843E-32));
#24410=DIRECTION('',(6.02124417213198E-17,-1.,2.60927675461843E-32));
#24411=DIRECTION('',(-0.707106781186546,-4.25766258529449E-17,-0.707106781186549));
#24412=DIRECTION('center_axis',(-1.02201073032319E-15,-0.713250449154181,
0.700909264299851));
#24413=DIRECTION('ref_axis',(-1.,-6.02124417213166E-17,-1.51939392966847E-15));
#24414=DIRECTION('center_axis',(6.02124417213198E-17,-1.,2.60927675461843E-32));
#24415=DIRECTION('ref_axis',(-1.,-6.02124417213198E-17,-1.51939392966847E-15));
#24416=DIRECTION('center_axis',(-6.02124417213198E-17,1.,-2.60927675461843E-32));
#24417=DIRECTION('ref_axis',(-1.,-6.02124417213198E-17,-1.51939392966847E-15));
#24418=DIRECTION('',(-0.707106781186546,0.707106781186549,-1.1609693565858E-15));
#24419=DIRECTION('center_axis',(6.02124417213198E-17,-1.,2.60927675461843E-32));
#24420=DIRECTION('ref_axis',(-1.,-6.02124417213198E-17,-1.51939392966847E-15));
#24421=DIRECTION('center_axis',(-6.02124417213198E-17,1.,-2.60927675461843E-32));
#24422=DIRECTION('ref_axis',(-1.51939392966847E-15,-6.53936508957055E-32,
1.));
#24423=DIRECTION('center_axis',(-6.02124417213198E-17,1.,-2.60927675461843E-32));
#24424=DIRECTION('ref_axis',(-1.,-6.02124417213198E-17,-1.51939392966847E-15));
#24425=DIRECTION('center_axis',(6.02124417213198E-17,-1.,2.60927675461843E-32));
#24426=DIRECTION('ref_axis',(-1.,-6.02124417213198E-17,-1.51939392966847E-15));
#24427=DIRECTION('center_axis',(-6.02124417213198E-17,1.,-2.60927675461843E-32));
#24428=DIRECTION('ref_axis',(-1.,-6.02124417213198E-17,-1.51939392966847E-15));
#24429=DIRECTION('',(-6.02124417213198E-17,1.,-2.60927675461843E-32));
#24430=DIRECTION('center_axis',(-6.02124417213198E-17,1.,-2.60927675461843E-32));
#24431=DIRECTION('ref_axis',(-1.,-6.02124417213198E-17,-1.51939392966847E-15));
#24432=DIRECTION('center_axis',(6.02124417213198E-17,-1.,2.60927675461843E-32));
#24433=DIRECTION('ref_axis',(-1.,-6.02124417213198E-17,-1.51939392966847E-15));
#24434=DIRECTION('',(0.242535625036333,0.970142500145332,3.38805108720557E-16));
#24435=DIRECTION('center_axis',(6.02124417213198E-17,-1.,2.60927675461843E-32));
#24436=DIRECTION('ref_axis',(-1.,-6.02124417213198E-17,-1.51939392966847E-15));
#24437=DIRECTION('center_axis',(6.02124417213198E-17,-1.,2.60927675461843E-32));
#24438=DIRECTION('ref_axis',(1.,6.02124417213198E-17,1.51939392966847E-15));
#24439=DIRECTION('',(6.02124417213198E-17,-1.,2.60927675461843E-32));
#24440=DIRECTION('center_axis',(6.02124417213198E-17,-1.,2.60927675461843E-32));
#24441=DIRECTION('ref_axis',(1.,6.02124417213198E-17,1.51939392966847E-15));
#24442=DIRECTION('center_axis',(6.02124417213198E-17,-1.,2.60927675461843E-32));
#24443=DIRECTION('ref_axis',(1.,6.02124417213198E-17,1.51939392966847E-15));
#24444=DIRECTION('center_axis',(6.02124417213198E-17,-1.,2.60927675461843E-32));
#24445=DIRECTION('ref_axis',(1.,6.02124417213198E-17,1.51939392966847E-15));
#24446=DIRECTION('center_axis',(6.02124417213198E-17,-1.,2.60927675461843E-32));
#24447=DIRECTION('ref_axis',(1.,6.02124417213198E-17,1.51939392966847E-15));
#24448=DIRECTION('',(6.02124417213198E-17,-1.,2.60927675461843E-32));
#24449=DIRECTION('center_axis',(6.02124417213198E-17,-1.,2.60927675461843E-32));
#24450=DIRECTION('ref_axis',(1.,6.02124417213198E-17,1.51939392966847E-15));
#24451=DIRECTION('center_axis',(6.02124417213198E-17,-1.,2.60927675461843E-32));
#24452=DIRECTION('ref_axis',(1.,6.02124417213198E-17,1.51939392966847E-15));
#24453=DIRECTION('center_axis',(6.02124417213198E-17,-1.,2.60927675461843E-32));
#24454=DIRECTION('ref_axis',(1.,6.02124417213198E-17,1.51939392966847E-15));
#24455=DIRECTION('',(6.02124417213198E-17,-1.,2.60927675461843E-32));
#24456=DIRECTION('center_axis',(6.02124417213198E-17,-1.,2.60927675461843E-32));
#24457=DIRECTION('ref_axis',(1.,6.02124417213198E-17,1.51939392966847E-15));
#24458=DIRECTION('center_axis',(6.02124417213198E-17,-1.,2.60927675461843E-32));
#24459=DIRECTION('ref_axis',(1.,6.02124417213198E-17,1.51939392966847E-15));
#24460=DIRECTION('center_axis',(6.02124417213198E-17,-1.,2.60927675461843E-32));
#24461=DIRECTION('ref_axis',(1.,6.02124417213198E-17,1.51939392966847E-15));
#24462=DIRECTION('',(6.02124417213198E-17,-1.,2.60927675461843E-32));
#24463=DIRECTION('center_axis',(6.02124417213198E-17,-1.,2.60927675461843E-32));
#24464=DIRECTION('ref_axis',(1.,6.02124417213198E-17,1.51939392966847E-15));
#24465=DIRECTION('center_axis',(6.02124417213198E-17,-1.,2.60927675461843E-32));
#24466=DIRECTION('ref_axis',(1.,6.02124417213198E-17,1.51939392966847E-15));
#24467=DIRECTION('center_axis',(6.02124417213198E-17,-1.,2.60927675461843E-32));
#24468=DIRECTION('ref_axis',(1.,6.02124417213198E-17,1.51939392966847E-15));
#24469=DIRECTION('',(6.02124417213198E-17,-1.,2.60927675461843E-32));
#24470=DIRECTION('center_axis',(-6.02124417213198E-17,1.,-2.60927675461843E-32));
#24471=DIRECTION('ref_axis',(-1.51939392966847E-15,-6.53936508957055E-32,
1.));
#24472=DIRECTION('',(1.,6.02124417213198E-17,1.51939392966847E-15));
#24473=DIRECTION('',(1.00165684600473E-12,6.02861116972749E-29,-1.));
#24474=DIRECTION('',(-1.,-6.02124417213198E-17,-1.00165684600473E-12));
#24475=DIRECTION('center_axis',(6.02124417213198E-17,-1.,2.60927675461843E-32));
#24476=DIRECTION('ref_axis',(1.,6.02124417213198E-17,1.51939392966847E-15));
#24477=DIRECTION('center_axis',(6.02124417213198E-17,-1.,2.60927675461843E-32));
#24478=DIRECTION('ref_axis',(1.,6.02124417213198E-17,1.51939392966847E-15));
#24479=DIRECTION('',(6.02124417213198E-17,-1.,2.60927675461843E-32));
#24480=DIRECTION('center_axis',(6.02124417213198E-17,-1.,2.60927675461843E-32));
#24481=DIRECTION('ref_axis',(1.,6.02124417213198E-17,1.51939392966847E-15));
#24482=DIRECTION('center_axis',(-6.02124417213198E-17,1.,-2.60927675461843E-32));
#24483=DIRECTION('ref_axis',(-1.51939392966847E-15,-6.53936508957055E-32,
1.));
#24484=DIRECTION('center_axis',(-6.02124417213198E-17,1.,-2.60927675461843E-32));
#24485=DIRECTION('ref_axis',(-1.51939392966847E-15,-6.53936508957055E-32,
1.));
#24486=DIRECTION('center_axis',(1.51939392966847E-15,6.53936508957056E-32,
-1.));
#24487=DIRECTION('ref_axis',(1.,6.02124417213198E-17,1.51939392966847E-15));
#24488=DIRECTION('center_axis',(-1.,-6.02124417213198E-17,-1.6568460057356E-15));
#24489=DIRECTION('ref_axis',(6.02124417213198E-17,-1.,2.60927675461843E-32));
#24490=DIRECTION('center_axis',(-1.6568460057356E-15,-7.36699760153718E-32,
1.));
#24491=DIRECTION('ref_axis',(-1.,-6.02124417213198E-17,-1.6568460057356E-15));
#24492=DIRECTION('center_axis',(0.999847695156391,-0.0174524064372835,1.51916251861363E-15));
#24493=DIRECTION('ref_axis',(-1.51939392966847E-15,-9.04549301518072E-32,
1.));
#30302=CARTESIAN_POINT('',(0.,0.,0.));
#30303=CARTESIAN_POINT('Origin',(-0.0129631448730623,-0.024,0.02115));
#30304=CARTESIAN_POINT('',(0.0129631448730622,-0.0244065057546663,0.0211500000000126));
#30305=CARTESIAN_POINT('',(-0.0129631448730623,-0.0244065057553825,0.02115));
#30306=CARTESIAN_POINT('',(0.00151842756346932,-0.0244065057553835,0.02115));
#30307=CARTESIAN_POINT('',(0.0129631448730622,-0.024,0.0211500000000126));
#30308=CARTESIAN_POINT('',(0.0129631448730622,-0.024,0.0211500000000126));
#30309=CARTESIAN_POINT('',(-0.0129631448730623,-0.024,0.02115));
#30310=CARTESIAN_POINT('',(-0.00648157243653117,-0.024,0.02115));
#30311=CARTESIAN_POINT('',(-0.0129631448730623,-0.024,0.02115));
#30312=CARTESIAN_POINT('Origin',(-0.0129631448730724,-0.024,0.0191500000000103));
#30313=CARTESIAN_POINT('',(-0.0137123694637994,-0.0327500380762009,0.0210043631016193));
#30314=CARTESIAN_POINT('Origin',(-0.0129631448730724,-0.138986429016312,
0.0191500000000103));
#30315=CARTESIAN_POINT('',(-0.0140842817269636,-0.024,0.0208062162162381));
#30316=CARTESIAN_POINT('Origin',(-0.0129631448730724,-0.024,0.0191500000000103));
#30317=CARTESIAN_POINT('',(-0.0140842817269636,-0.0329447564781601,0.0208062162162381));
#30318=CARTESIAN_POINT('',(-0.0140842817269636,-0.024,0.0208062162162381));
#30319=CARTESIAN_POINT('Origin',(-0.0129631448730724,-0.034572315620975,
0.0191500000000103));
#30320=CARTESIAN_POINT('Origin',(-1.00275343584144E-14,-0.024,9.9475983006414E-15));
#30321=CARTESIAN_POINT('',(-0.0141669730359352,-0.033,0.02075000000001));
#30322=CARTESIAN_POINT('Origin',(-1.00275343584144E-14,-0.0533909682096408,
9.9475983006414E-15));
#30323=CARTESIAN_POINT('',(-0.0208062162162391,-0.024,0.0140842817269642));
#30324=CARTESIAN_POINT('Origin',(-1.00275343584144E-14,-0.024,9.9475983006414E-15));
#30325=CARTESIAN_POINT('',(-0.0208062162162391,-0.0329447564781591,0.0140842817269642));
#30326=CARTESIAN_POINT('',(-0.0208062162162391,-0.024,0.0140842817269642));
#30327=CARTESIAN_POINT('',(-0.0207500000000101,-0.033,0.014166973035935));
#30328=CARTESIAN_POINT('Origin',(-1.00275343584144E-14,-0.0533909682096407,
9.9475983006414E-15));
#30329=CARTESIAN_POINT('',(-0.0181707160081772,-0.033,0.017351965443474));
#30330=CARTESIAN_POINT('Origin',(-1.00275343584144E-14,-0.033,9.9475983006414E-15));
#30331=CARTESIAN_POINT('',(-0.017351965443474,-0.033,0.0181707160081772));
#30332=CARTESIAN_POINT('Ctrl Pts',(-0.0173519654434766,-0.0330000000000234,
0.0181707160081747));
#30333=CARTESIAN_POINT('Ctrl Pts',(-0.0175505715951354,-0.0329573203740106,
0.0179810588103573));
#30334=CARTESIAN_POINT('Ctrl Pts',(-0.017753450710576,-0.0329436053651554,
0.0177809667685882));
#30335=CARTESIAN_POINT('Ctrl Pts',(-0.0180265973873143,-0.0329719202135652,
0.0175019481550689));
#30336=CARTESIAN_POINT('Ctrl Pts',(-0.0180989364030346,-0.0329838470317312,
0.0174271319613231));
#30337=CARTESIAN_POINT('Ctrl Pts',(-0.0181707160081747,-0.0330000000000234,
0.0173519654434766));
#30338=CARTESIAN_POINT('Origin',(-1.00275343584144E-14,-0.033,9.9475983006414E-15));
#30339=CARTESIAN_POINT('Origin',(-0.0191500000000098,-0.024,0.0129631448730722));
#30340=CARTESIAN_POINT('',(-0.0210043631016193,-0.0327500380762009,0.0137123694638626));
#30341=CARTESIAN_POINT('Origin',(-0.0191500000000098,-0.0345723156209755,
0.0129631448730722));
#30342=CARTESIAN_POINT('',(-0.0211500000000238,-0.024,0.0129631448730623));
#30343=CARTESIAN_POINT('Origin',(-0.0191500000000098,-0.024,0.0129631448730722));
#30344=CARTESIAN_POINT('',(-0.0211500000000238,-0.0244065057540237,0.0129631448730623));
#30345=CARTESIAN_POINT('',(-0.0211500000000238,-0.024,0.0129631448730623));
#30346=CARTESIAN_POINT('Origin',(-0.0191500000000098,-0.138986429016342,
0.0129631448730722));
#30347=CARTESIAN_POINT('Origin',(-0.02115,-0.024,-0.0129631448730623));
#30348=CARTESIAN_POINT('',(-0.02115,-0.0244065057553841,-0.0129631448730623));
#30349=CARTESIAN_POINT('',(-0.02115,-0.0244065057553851,0.00151842756346924));
#30350=CARTESIAN_POINT('',(-0.02115,-0.024,-0.0129631448730623));
#30351=CARTESIAN_POINT('',(-0.02115,-0.024,-0.00648157243653115));
#30352=CARTESIAN_POINT('',(-0.02115,-0.024,-0.0129631448730623));
#30353=CARTESIAN_POINT('Origin',(-0.01915000000001,-0.024,-0.0129631448730723));
#30354=CARTESIAN_POINT('',(-0.0210043631016193,-0.0327500380762009,-0.0137123694637993));
#30355=CARTESIAN_POINT('Origin',(-0.01915000000001,-0.138986429016327,-0.0129631448730723));
#30356=CARTESIAN_POINT('',(-0.0208062162162194,-0.024,-0.0140842817269509));
#30357=CARTESIAN_POINT('Origin',(-0.01915000000001,-0.024,-0.0129631448730723));
#30358=CARTESIAN_POINT('',(-0.0208062162162194,-0.0329447564781784,-0.0140842817269509));
#30359=CARTESIAN_POINT('',(-0.0208062162162194,-0.024,-0.0140842817269509));
#30360=CARTESIAN_POINT('Origin',(-0.01915000000001,-0.0345723156209752,
-0.0129631448730723));
#30361=CARTESIAN_POINT('Origin',(-1.00275343584144E-14,-0.024,9.9475983006414E-15));
#30362=CARTESIAN_POINT('',(-0.0207500000000101,-0.033,-0.0141669730359174));
#30363=CARTESIAN_POINT('Origin',(-1.00275343584144E-14,-0.0533909682096407,
9.9475983006414E-15));
#30364=CARTESIAN_POINT('',(-0.014084281726955,-0.024,-0.0208062162162255));
#30365=CARTESIAN_POINT('Origin',(-1.00275343584144E-14,-0.024,9.9475983006414E-15));
#30366=CARTESIAN_POINT('',(-0.014084281726955,-0.0329447564781725,-0.0208062162162255));
#30367=CARTESIAN_POINT('',(-0.014084281726955,-0.024,-0.0208062162162255));
#30368=CARTESIAN_POINT('',(-0.0141669730359082,-0.033,-0.02075000000001));
#30369=CARTESIAN_POINT('Origin',(-1.00275343584144E-14,-0.0533909682096603,
9.9475983006414E-15));
#30370=CARTESIAN_POINT('',(-0.0173519654434044,-0.033,-0.0181707160082254));
#30371=CARTESIAN_POINT('Origin',(-1.00275343584144E-14,-0.033,9.9475983006414E-15));
#30372=CARTESIAN_POINT('',(-0.018170716008223,-0.033,-0.0173519654434079));
#30373=CARTESIAN_POINT('Ctrl Pts',(-0.0181707160082205,-0.0330000000000234,
-0.0173519654434105));
#30374=CARTESIAN_POINT('Ctrl Pts',(-0.0179810588103863,-0.0329573203740007,
-0.0175505715950879));
#30375=CARTESIAN_POINT('Ctrl Pts',(-0.0177809667685979,-0.0329436053651405,
-0.0177534507105486));
#30376=CARTESIAN_POINT('Ctrl Pts',(-0.0175019481550389,-0.0329719202135544,
-0.0180265973873254));
#30377=CARTESIAN_POINT('Ctrl Pts',(-0.0174271319612734,-0.0329838470317247,
-0.0180989364030644));
#30378=CARTESIAN_POINT('Ctrl Pts',(-0.0173519654434071,-0.0330000000000234,
-0.0181707160082229));
#30379=CARTESIAN_POINT('Origin',(-1.00275343584144E-14,-0.033,9.9475983006414E-15));
#30380=CARTESIAN_POINT('Origin',(-0.0129631448730721,-0.024,-0.0191500000000097));
#30381=CARTESIAN_POINT('',(-0.0137123694638186,-0.0327500380762009,-0.0210043631016193));
#30382=CARTESIAN_POINT('Origin',(-0.0129631448730721,-0.0345723156209755,
-0.0191500000000097));
#30383=CARTESIAN_POINT('',(-0.0129631448730622,-0.024,-0.0211500000000074));
#30384=CARTESIAN_POINT('Origin',(-0.0129631448730721,-0.024,-0.0191500000000097));
#30385=CARTESIAN_POINT('',(-0.0129631448730622,-0.0244065057549635,-0.0211500000000074));
#30386=CARTESIAN_POINT('',(-0.0129631448730622,-0.024,-0.0211500000000074));
#30387=CARTESIAN_POINT('Origin',(-0.0129631448730721,-0.138986429016347,
-0.0191500000000097));
#30388=CARTESIAN_POINT('Origin',(0.0129631448730622,-0.024,-0.0211500000000226));
#30389=CARTESIAN_POINT('',(0.0129631448730622,-0.0244065057540901,-0.0211500000000226));
#30390=CARTESIAN_POINT('',(-0.00151842756367382,-0.0244065057548141,-0.02115000000001));
#30391=CARTESIAN_POINT('',(0.0129631448730622,-0.024,-0.0211500000000226));
#30392=CARTESIAN_POINT('',(0.00648157243652186,-0.024,-0.0211500000000169));
#30393=CARTESIAN_POINT('',(0.0129631448730622,-0.024,-0.0211500000000226));
#30394=CARTESIAN_POINT('Origin',(0.012963144873072,-0.024,-0.0191500000000096));
#30395=CARTESIAN_POINT('',(0.0137123694638594,-0.0327500380762009,-0.0210043631016193));
#30396=CARTESIAN_POINT('Origin',(0.012963144873072,-0.138986429016351,-0.0191500000000096));
#30397=CARTESIAN_POINT('',(0.0140842817269635,-0.024,-0.0208062162162381));
#30398=CARTESIAN_POINT('Origin',(0.012963144873072,-0.024,-0.0191500000000096));
#30399=CARTESIAN_POINT('',(0.0140842817269635,-0.0329447564781601,-0.0208062162162381));
#30400=CARTESIAN_POINT('',(0.0140842817269635,-0.024,-0.0208062162162381));
#30401=CARTESIAN_POINT('Origin',(0.012963144873072,-0.0345723156209756,
-0.0191500000000096));
#30402=CARTESIAN_POINT('Origin',(-1.00275343584144E-14,-0.024,9.9475983006414E-15));
#30403=CARTESIAN_POINT('',(0.0141669730358882,-0.033,-0.02075000000001));
#30404=CARTESIAN_POINT('Origin',(-1.00275343584144E-14,-0.0533909682096603,
9.9475983006414E-15));
#30405=CARTESIAN_POINT('',(0.0208062162162161,-0.024,-0.0140842817269487));
#30406=CARTESIAN_POINT('Origin',(-1.00275343584144E-14,-0.024,9.9475983006414E-15));
#30407=CARTESIAN_POINT('',(0.0208062162162161,-0.0329447564781817,-0.0140842817269487));
#30408=CARTESIAN_POINT('',(0.0208062162162161,-0.024,-0.0140842817269487));
#30409=CARTESIAN_POINT('',(0.02075000000001,-0.033,-0.0141669730358881));
#30410=CARTESIAN_POINT('Origin',(-1.00275343584144E-14,-0.0533909682096601,
9.9475983006414E-15));
#30411=CARTESIAN_POINT('',(0.0181707160082761,-0.033,-0.0173519654433313));
#30412=CARTESIAN_POINT('Origin',(-1.00275343584144E-14,-0.033,9.9475983006414E-15));
#30413=CARTESIAN_POINT('',(0.0173519654433313,-0.033,-0.0181707160082761));
#30414=CARTESIAN_POINT('Ctrl Pts',(0.0173519654433339,-0.0330000000000234,
-0.0181707160082736));
#30415=CARTESIAN_POINT('Ctrl Pts',(0.0175505715950326,-0.0329573203739897,
-0.0179810588104207));
#30416=CARTESIAN_POINT('Ctrl Pts',(0.0177534507105162,-0.0329436053651239,
-0.0177809667686107));
#30417=CARTESIAN_POINT('Ctrl Pts',(0.0180265973873359,-0.0329719202135427,
-0.0175019481550082));
#30418=CARTESIAN_POINT('Ctrl Pts',(0.0180989364030953,-0.0329838470317177,
-0.0174271319612215));
#30419=CARTESIAN_POINT('Ctrl Pts',(0.0181707160082736,-0.0330000000000234,
-0.0173519654433339));
#30420=CARTESIAN_POINT('Origin',(-1.00275343584144E-14,-0.033,9.9475983006414E-15));
#30421=CARTESIAN_POINT('Origin',(0.0211500000000181,-0.024,-0.00793218971944487));
#30422=CARTESIAN_POINT('',(0.0211500000000181,-0.031,-0.00793218971944487));
#30423=CARTESIAN_POINT('',(0.0211500000000182,-0.03099999999999,-0.00800000000000997));
#30424=CARTESIAN_POINT('',(0.0211500000000147,-0.031,-0.00396609485971326));
#30425=CARTESIAN_POINT('',(0.0211500000000181,-0.0328178102805551,-0.00793218971944487));
#30426=CARTESIAN_POINT('',(0.0211500000000181,-0.024,-0.00793218971944487));
#30427=CARTESIAN_POINT('',(0.0211500000000182,-0.03274999999999,-0.00800000000000997));
#30428=CARTESIAN_POINT('',(0.02115000000002,-0.0306419525701411,-0.0101080474298589));
#30429=CARTESIAN_POINT('',(0.0211500000000182,-0.0283771628421106,-0.008));
#30430=CARTESIAN_POINT('Origin',(0.02115,-0.024,0.0129631448730622));
#30431=CARTESIAN_POINT('',(0.0211500000000043,-0.03099999999999,0.00800000000001003));
#30432=CARTESIAN_POINT('',(0.0211500000000044,-0.031,0.00793218971944469));
#30433=CARTESIAN_POINT('',(0.0211500000000056,-0.031,0.00648157243654025));
#30434=CARTESIAN_POINT('',(0.0211500000000043,-0.03274999999999,0.00800000000001004));
#30435=CARTESIAN_POINT('',(0.0211500000000043,-0.0285,0.008));
#30436=CARTESIAN_POINT('',(0.0211500000000044,-0.0328178102805553,0.00793218971944469));
#30437=CARTESIAN_POINT('',(0.0211500000000014,-0.0293842137817322,0.0113657862182679));
#30438=CARTESIAN_POINT('',(0.0211500000000044,-0.024,0.00793218971944469));
#30439=CARTESIAN_POINT('Origin',(0.0211500000000044,-0.024,0.00793218971944473));
#30440=CARTESIAN_POINT('',(0.0248178102805753,-0.03099999999999,0.00793218971944473));
#30441=CARTESIAN_POINT('',(0.0105750000000022,-0.031,0.00793218971944473));
#30442=CARTESIAN_POINT('',(0.02475000000001,-0.0328178102805653,0.00793218971944473));
#30443=CARTESIAN_POINT('',(0.0158250000000022,-0.0328178102805553,0.00793218971944473));
#30444=CARTESIAN_POINT('',(0.0248178102805753,-0.03274999999999,0.00793218971944473));
#30445=CARTESIAN_POINT('',(0.0261339051402787,-0.0314339051402766,0.00793218971944473));
#30446=CARTESIAN_POINT('',(0.0248178102805553,-0.0285,0.00793218971944473));
#30447=CARTESIAN_POINT('Origin',(0.02115,-0.024,0.0129631448730622));
#30448=CARTESIAN_POINT('',(0.0211500000000043,-0.0244065057561963,0.00800000000001003));
#30449=CARTESIAN_POINT('',(0.02115,-0.0244065057553837,0.0129631448730622));
#30450=CARTESIAN_POINT('',(0.0211500000000126,-0.0244065057546653,-0.00151842756326574));
#30451=CARTESIAN_POINT('',(0.0211500000000043,-0.02399999999999,0.00800000000000138));
#30452=CARTESIAN_POINT('',(0.0211500000000043,-0.024,0.008));
#30453=CARTESIAN_POINT('',(0.02115,-0.024,0.0129631448730622));
#30454=CARTESIAN_POINT('',(0.0211500000000056,-0.024,0.00648157243654025));
#30455=CARTESIAN_POINT('',(0.02115,-0.024,0.0129631448730622));
#30456=CARTESIAN_POINT('Origin',(0.01915000000001,-0.024,0.0129631448730722));
#30457=CARTESIAN_POINT('',(0.0210043631016192,-0.0327500380762009,0.0137123694637995));
#30458=CARTESIAN_POINT('',(0.020806216216238,-0.0329447564781601,0.0140842817269634));
#30459=CARTESIAN_POINT('Origin',(0.01915000000001,-0.0345723156209752,0.0129631448730722));
#30460=CARTESIAN_POINT('Origin',(0.01915000000001,-0.138986429016329,0.0129631448730722));
#30461=CARTESIAN_POINT('',(0.020806216216238,-0.024,0.0140842817269634));
#30462=CARTESIAN_POINT('Origin',(0.01915000000001,-0.024,0.0129631448730722));
#30463=CARTESIAN_POINT('',(0.020806216216238,-0.024,0.0140842817269634));
#30464=CARTESIAN_POINT('Origin',(-1.00275343584144E-14,-0.024,9.9475983006414E-15));
#30465=CARTESIAN_POINT('',(0.0141669730359443,-0.033,0.02075000000001));
#30466=CARTESIAN_POINT('',(0.014084281726958,-0.0329447564781683,0.0208062162162298));
#30467=CARTESIAN_POINT('Origin',(-1.00275343584144E-14,-0.0533909682096408,
9.9475983006414E-15));
#30468=CARTESIAN_POINT('',(0.017351965443488,-0.033,0.0181707160081675));
#30469=CARTESIAN_POINT('Origin',(-1.00275343584144E-14,-0.033,9.9475983006414E-15));
#30470=CARTESIAN_POINT('',(0.0181707160081698,-0.033,0.0173519654434845));
#30471=CARTESIAN_POINT('Ctrl Pts',(0.0181707160081673,-0.0330000000000234,
0.0173519654434871));
#30472=CARTESIAN_POINT('Ctrl Pts',(0.017981058810353,-0.0329573203740124,
0.0175505715951428));
#30473=CARTESIAN_POINT('Ctrl Pts',(0.0177809667685874,-0.0329436053651581,
0.0177534507105799));
#30474=CARTESIAN_POINT('Ctrl Pts',(0.0175019481550755,-0.0329719202135672,
0.0180265973873114));
#30475=CARTESIAN_POINT('Ctrl Pts',(0.0174271319613334,-0.0329838470317324,
0.0180989364030283));
#30476=CARTESIAN_POINT('Ctrl Pts',(0.0173519654434906,-0.0330000000000234,
0.0181707160081649));
#30477=CARTESIAN_POINT('',(0.02075000000001,-0.033,0.0141669730359351));
#30478=CARTESIAN_POINT('Origin',(-1.00275343584144E-14,-0.033,9.9475983006414E-15));
#30479=CARTESIAN_POINT('Origin',(-1.00275343584144E-14,-0.0533909682096601,
9.9475983006414E-15));
#30480=CARTESIAN_POINT('',(0.014084281726958,-0.024,0.0208062162162298));
#30481=CARTESIAN_POINT('Origin',(-1.00275343584144E-14,-0.024,9.9475983006414E-15));
#30482=CARTESIAN_POINT('',(0.014084281726958,-0.024,0.0208062162162298));
#30483=CARTESIAN_POINT('Origin',(0.0129631448730721,-0.024,0.0191500000000096));
#30484=CARTESIAN_POINT('',(0.0137123694638326,-0.0327500380762009,0.0210043631016193));
#30485=CARTESIAN_POINT('Origin',(0.0129631448730721,-0.138986429016353,
0.0191500000000096));
#30486=CARTESIAN_POINT('Origin',(0.0129631448730721,-0.0345723156209757,
0.0191500000000096));
#30487=CARTESIAN_POINT('Origin',(0.0129631448730721,-0.024,0.0191500000000096));
#30488=CARTESIAN_POINT('Origin',(0.01915000000001,-0.024,-0.0129631448730722));
#30489=CARTESIAN_POINT('',(0.0211500000000225,-0.024,-0.0129631448730622));
#30490=CARTESIAN_POINT('Origin',(0.01915000000001,-0.024,-0.0129631448730722));
#30491=CARTESIAN_POINT('',(0.0211500000000225,-0.0244065057540974,-0.0129631448730622));
#30492=CARTESIAN_POINT('',(0.0211500000000225,-0.024,-0.0129631448730622));
#30493=CARTESIAN_POINT('',(0.0210043631016192,-0.0327500380762009,-0.0137123694637889));
#30494=CARTESIAN_POINT('Origin',(0.01915000000001,-0.13898642901633,-0.0129631448730722));
#30495=CARTESIAN_POINT('Origin',(0.01915000000001,-0.0345723156209752,-0.0129631448730722));
#30496=CARTESIAN_POINT('Origin',(0.0211500000000181,-0.024,-0.00793218971944487));
#30497=CARTESIAN_POINT('',(0.0211500000000182,-0.02399999999999,-0.00800000000002138));
#30498=CARTESIAN_POINT('',(0.0211500000000147,-0.024,-0.00396609485971326));
#30499=CARTESIAN_POINT('',(0.0211500000000182,-0.0244065057553889,-0.00800000000000997));
#30500=CARTESIAN_POINT('',(0.0211500000000182,-0.024,-0.008));
#30501=CARTESIAN_POINT('',(0.0211500000000216,-0.0244065057541469,-0.0119660948595193));
#30502=CARTESIAN_POINT('Origin',(0.02715,-0.024,-0.00793218971944484));
#30503=CARTESIAN_POINT('',(0.0248178102805751,-0.03099999999999,-0.00793218971944484));
#30504=CARTESIAN_POINT('',(0.013575,-0.031,-0.00793218971944483));
#30505=CARTESIAN_POINT('',(0.0248178102805751,-0.03274999999999,-0.00793218971944484));
#30506=CARTESIAN_POINT('',(0.0248178102805552,-0.0284385814210553,-0.00793218971944484));
#30507=CARTESIAN_POINT('',(0.0247500000000101,-0.0328178102805551,-0.00793218971944484));
#30508=CARTESIAN_POINT('',(0.0275714051402776,-0.0299964051402776,-0.00793218971944484));
#30509=CARTESIAN_POINT('',(0.018825,-0.0328178102805552,-0.00793218971944484));
#30510=CARTESIAN_POINT('Origin',(0.016,-0.033,0.021));
#30511=CARTESIAN_POINT('',(0.00800000000000993,-0.0327500380762009,0.0210043631016193));
#30512=CARTESIAN_POINT('Origin',(-0.0155,-0.032875,0.0155));
#30513=CARTESIAN_POINT('',(-0.01850000000002,-0.03274999999999,0.01550000000001));
#30514=CARTESIAN_POINT('',(-0.0125000000000076,-0.0327499999999924,0.0155));
#30515=CARTESIAN_POINT('Origin',(-0.01550000000001,-0.03274999999999,0.01550000000001));
#30516=CARTESIAN_POINT('',(-0.0122499999999766,-0.0330000000000234,0.0155));
#30517=CARTESIAN_POINT('',(-0.012375,-0.032875,0.0155));
#30518=CARTESIAN_POINT('Origin',(-0.01550000000001,-0.033,0.01550000000001));
#30519=CARTESIAN_POINT('Origin',(-0.01550000000001,-0.033,0.01550000000001));
#30520=CARTESIAN_POINT('Origin',(-0.01550000000001,-0.03274999999999,0.01550000000001));
#30521=CARTESIAN_POINT('Origin',(-0.021,-0.033,0.016));
#30522=CARTESIAN_POINT('',(-0.0210043631016193,-0.0327500380762009,0.00800000000000997));
#30523=CARTESIAN_POINT('Origin',(-0.0208771815508047,-0.0328750190381054,
0.008));
#30524=CARTESIAN_POINT('',(-0.0207500000000101,-0.033,0.00800000000000997));
#30525=CARTESIAN_POINT('Origin',(-0.0155,-0.032875,-0.0155));
#30526=CARTESIAN_POINT('',(-0.01850000000002,-0.03274999999999,-0.0155000000000101));
#30527=CARTESIAN_POINT('',(-0.0125000000000076,-0.0327499999999924,-0.0155));
#30528=CARTESIAN_POINT('Origin',(-0.01550000000001,-0.03274999999999,-0.01550000000001));
#30529=CARTESIAN_POINT('',(-0.0122499999999766,-0.0330000000000234,-0.0155));
#30530=CARTESIAN_POINT('',(-0.012375,-0.032875,-0.0155));
#30531=CARTESIAN_POINT('Origin',(-0.01550000000001,-0.033,-0.01550000000001));
#30532=CARTESIAN_POINT('Origin',(-0.01550000000001,-0.033,-0.01550000000001));
#30533=CARTESIAN_POINT('Origin',(-0.01550000000001,-0.03274999999999,-0.01550000000001));
#30534=CARTESIAN_POINT('Origin',(-0.016,-0.033,-0.021));
#30535=CARTESIAN_POINT('',(-0.00800000000001002,-0.0327500380762009,-0.0210043631016193));
#30536=CARTESIAN_POINT('Origin',(-0.008,-0.0328750190381054,-0.0208771815508047));
#30537=CARTESIAN_POINT('',(-0.00800000000001002,-0.033,-0.02075000000001));
#30538=CARTESIAN_POINT('Origin',(0.0155,-0.032875,-0.0155));
#30539=CARTESIAN_POINT('',(0.0125,-0.03274999999999,-0.01550000000001));
#30540=CARTESIAN_POINT('',(0.0184999999999924,-0.0327499999999924,-0.0155));
#30541=CARTESIAN_POINT('Origin',(0.01550000000001,-0.03274999999999,-0.01550000000001));
#30542=CARTESIAN_POINT('',(0.0187500000000234,-0.0330000000000234,-0.0155));
#30543=CARTESIAN_POINT('',(0.018625,-0.032875,-0.0155));
#30544=CARTESIAN_POINT('Origin',(0.01550000000001,-0.033,-0.01550000000001));
#30545=CARTESIAN_POINT('Origin',(0.01550000000001,-0.033,-0.01550000000001));
#30546=CARTESIAN_POINT('Origin',(0.01550000000001,-0.03274999999999,-0.01550000000001));
#30547=CARTESIAN_POINT('Origin',(0.0208771815508047,-0.0328750190381054,
-0.008));
#30548=CARTESIAN_POINT('',(0.0210043631016093,-0.0327500380762109,-0.00799996192378907));
#30549=CARTESIAN_POINT('',(0.0210043631016192,-0.0327500380762009,-0.01200000000001));
#30550=CARTESIAN_POINT('',(0.02075,-0.033,-0.00775));
#30551=CARTESIAN_POINT('',(0.0191281314609001,-0.0345938057745268,-0.00615619422549322));
#30552=CARTESIAN_POINT('',(0.02075000000001,-0.033,-0.00800000000000997));
#30553=CARTESIAN_POINT('Origin',(0.021,-0.0327543256842211,-0.008));
#30554=CARTESIAN_POINT('',(0.021004363766232,-0.03275,-0.008));
#30555=CARTESIAN_POINT('',(0.01050000000001,-0.03274999999999,-0.00800000000000999));
#30556=CARTESIAN_POINT('',(0.0210349101298563,-0.031,-0.008));
#30557=CARTESIAN_POINT('',(0.0210006091729909,-0.0329651005032875,-0.00800000000000997));
#30558=CARTESIAN_POINT('',(0.0216250000000099,-0.03099999999999,-0.00800000000000997));
#30559=CARTESIAN_POINT('Origin',(0.0105,-0.032875,-0.007875));
#30560=CARTESIAN_POINT('',(0.02475,-0.033,-0.00775));
#30561=CARTESIAN_POINT('',(0.02475000000001,-0.03274999999999,-0.00800000000000996));
#30562=CARTESIAN_POINT('',(0.01050000000001,-0.033,-0.00775000000000998));
#30563=CARTESIAN_POINT('',(0.0210362867019386,-0.0309211362387957,-0.0098288637612043));
#30564=CARTESIAN_POINT('Origin',(0.024875,-0.033,0.007875));
#30565=CARTESIAN_POINT('',(0.025,-0.03275,0.00775));
#30566=CARTESIAN_POINT('',(0.02475000000001,-0.03274999999999,0.00800000000001004));
#30567=CARTESIAN_POINT('',(0.025,-0.031,0.00775));
#30568=CARTESIAN_POINT('',(0.02500000000001,-0.033,0.00775000000001004));
#30569=CARTESIAN_POINT('',(0.02062500000001,-0.03099999999999,0.01212500000001));
#30570=CARTESIAN_POINT('Origin',(-4.25999877636044E-17,-0.033,4.01748489384999E-31));
#30571=CARTESIAN_POINT('',(0.00800000000000993,-0.033,0.02075000000001));
#30572=CARTESIAN_POINT('',(0.02475,-0.033,0.00775));
#30573=CARTESIAN_POINT('',(0.02475000000001,-0.033,0.00400000000001004));
#30574=CARTESIAN_POINT('',(0.02075,-0.033,0.00775));
#30575=CARTESIAN_POINT('',(0.0105000000000099,-0.033,0.00775000000001002));
#30576=CARTESIAN_POINT('',(0.02075000000001,-0.033,-0.00800000000000997));
#30577=CARTESIAN_POINT('',(0.0187500000000234,-0.0330000000000234,0.0155));
#30578=CARTESIAN_POINT('Origin',(0.01550000000001,-0.033,0.01550000000001));
#30579=CARTESIAN_POINT('Origin',(0.01550000000001,-0.033,0.01550000000001));
#30580=CARTESIAN_POINT('',(-0.00450000000000004,-0.033,-7.38836374312403E-18));
#30581=CARTESIAN_POINT('Origin',(-4.48204338128547E-17,-0.033,3.98374757136611E-31));
#30582=CARTESIAN_POINT('Origin',(-0.0155,-0.03175,-0.0155));
#30583=CARTESIAN_POINT('',(-0.0185,-0.03049999999999,-0.0155));
#30584=CARTESIAN_POINT('Origin',(-0.01550000000001,-0.03049999999999,-0.01550000000001));
#30585=CARTESIAN_POINT('',(-0.0185,-0.03175,-0.0155));
#30586=CARTESIAN_POINT('Origin',(0.0155,-0.03175,-0.0155));
#30587=CARTESIAN_POINT('',(0.0125,-0.03049999999999,-0.0155));
#30588=CARTESIAN_POINT('Origin',(0.01550000000001,-0.03049999999999,-0.01550000000001));
#30589=CARTESIAN_POINT('',(0.0125,-0.03175,-0.0155));
#30590=CARTESIAN_POINT('Origin',(0.0155,-0.032875,0.0155));
#30591=CARTESIAN_POINT('',(0.0125,-0.03274999999999,0.01550000000001));
#30592=CARTESIAN_POINT('',(0.0184999999999924,-0.0327499999999924,0.0155));
#30593=CARTESIAN_POINT('Origin',(0.01550000000001,-0.03274999999999,0.01550000000001));
#30594=CARTESIAN_POINT('',(0.018625,-0.032875,0.0155));
#30595=CARTESIAN_POINT('Origin',(0.01550000000001,-0.03274999999999,0.01550000000001));
#30596=CARTESIAN_POINT('Origin',(0.0155,-0.03175,0.0155));
#30597=CARTESIAN_POINT('',(0.0125,-0.03049999999999,0.0155));
#30598=CARTESIAN_POINT('Origin',(0.01550000000001,-0.03049999999999,0.01550000000001));
#30599=CARTESIAN_POINT('',(0.0125,-0.03175,0.0155));
#30600=CARTESIAN_POINT('Origin',(-0.0155,-0.03175,0.0155));
#30601=CARTESIAN_POINT('',(-0.0185,-0.03049999999999,0.0155));
#30602=CARTESIAN_POINT('Origin',(-0.01550000000001,-0.03049999999999,0.01550000000001));
#30603=CARTESIAN_POINT('',(-0.0185,-0.03175,0.0155));
#30604=CARTESIAN_POINT('Origin',(0.0204055915910216,-0.024,0.01));
#30605=CARTESIAN_POINT('',(0.0189913780286485,-0.024,0.00858578643762694));
#30606=CARTESIAN_POINT('',(0.0204055915910216,-0.024,0.008));
#30607=CARTESIAN_POINT('Origin',(0.0204055915910316,-0.02399999999999,0.01000000000001));
#30608=CARTESIAN_POINT('',(0.0204055915910216,-0.031,0.008));
#30609=CARTESIAN_POINT('',(0.0204055915910316,-0.02399999999999,0.00800000000001003));
#30610=CARTESIAN_POINT('',(0.0189913780286485,-0.031,0.00858578643762694));
#30611=CARTESIAN_POINT('Origin',(0.0204055915910316,-0.03099999999999,0.01000000000001));
#30612=CARTESIAN_POINT('',(0.0189913780286585,-0.02399999999999,0.00858578643763693));
#30613=CARTESIAN_POINT('Origin',(0.025,-0.024,0.008));
#30614=CARTESIAN_POINT('',(0.0210349101298563,-0.031,0.008));
#30615=CARTESIAN_POINT('',(0.02100000000001,-0.033,0.00800000000001003));
#30616=CARTESIAN_POINT('',(0.02362500000001,-0.03099999999999,0.00800000000001004));
#30617=CARTESIAN_POINT('',(0.0125000000000099,-0.02399999999999,0.00800000000001002));
#30618=CARTESIAN_POINT('Origin',(-4.31418997390962E-17,-0.024,4.01513654477083E-31));
#30619=CARTESIAN_POINT('',(0.00807716446627529,-0.024,0.0195));
#30620=CARTESIAN_POINT('',(0.0166442911165788,-0.02399999999999,0.0109328733497165));
#30621=CARTESIAN_POINT('',(-0.00807716446627543,-0.024,0.0195));
#30622=CARTESIAN_POINT('',(0.0040385822331476,-0.02399999999999,0.01950000000001));
#30623=CARTESIAN_POINT('',(-0.0195,-0.024,0.00807716446627533));
#30624=CARTESIAN_POINT('',(-0.0109328733497166,-0.02399999999999,0.0166442911165788));
#30625=CARTESIAN_POINT('',(-0.0195,-0.024,-0.00807716446627539));
#30626=CARTESIAN_POINT('',(-0.0195000000000101,-0.02399999999999,0.00403858223314765));
#30627=CARTESIAN_POINT('',(-0.00807716446627538,-0.024,-0.0195));
#30628=CARTESIAN_POINT('',(-0.0166442911165788,-0.02399999999999,-0.0109328733497165));
#30629=CARTESIAN_POINT('',(0.00807716446627534,-0.024,-0.0195));
#30630=CARTESIAN_POINT('',(-0.00403858223314769,-0.02399999999999,-0.01950000000001));
#30631=CARTESIAN_POINT('',(0.0189913780286485,-0.024,-0.00858578643762688));
#30632=CARTESIAN_POINT('',(0.0109328733497165,-0.02399999999999,-0.0166442911165789));
#30633=CARTESIAN_POINT('',(0.0204055915910216,-0.024,-0.008));
#30634=CARTESIAN_POINT('Origin',(0.0204055915910316,-0.02399999999999,-0.01000000000001));
#30635=CARTESIAN_POINT('',(0.00975000000000998,-0.02399999999999,-0.00800000000000999));
#30636=CARTESIAN_POINT('',(0.0138,-0.02399999999999,-0.0155));
#30637=CARTESIAN_POINT('Origin',(0.01550000000001,-0.02399999999999,-0.01550000000001));
#30638=CARTESIAN_POINT('',(-0.0172,-0.02399999999999,0.0155));
#30639=CARTESIAN_POINT('Origin',(-0.01550000000001,-0.02399999999999,0.01550000000001));
#30640=CARTESIAN_POINT('',(0.0138,-0.02399999999999,0.0155));
#30641=CARTESIAN_POINT('Origin',(0.01550000000001,-0.02399999999999,0.01550000000001));
#30642=CARTESIAN_POINT('',(-0.0172,-0.02399999999999,-0.0155));
#30643=CARTESIAN_POINT('Origin',(-0.01550000000001,-0.02399999999999,-0.01550000000001));
#30644=CARTESIAN_POINT('Origin',(0.0204055915910216,-0.024,-0.01));
#30645=CARTESIAN_POINT('',(0.0189913780286485,-0.031,-0.00858578643762688));
#30646=CARTESIAN_POINT('',(0.0189913780286585,-0.02399999999999,-0.00858578643763687));
#30647=CARTESIAN_POINT('',(0.0204055915910216,-0.031,-0.008));
#30648=CARTESIAN_POINT('Origin',(0.0204055915910316,-0.03099999999999,-0.01000000000001));
#30649=CARTESIAN_POINT('',(0.0204055915910316,-0.02399999999999,-0.00800000000000997));
#30650=CARTESIAN_POINT('Origin',(0.00807716446627534,-0.024,-0.0195));
#30651=CARTESIAN_POINT('',(0.00807716446627534,-0.031,-0.0195));
#30652=CARTESIAN_POINT('',(0.00807716446628534,-0.02399999999999,-0.01950000000001));
#30653=CARTESIAN_POINT('',(0.0120208152801713,-0.031,-0.0155563491861041));
#30654=CARTESIAN_POINT('',(0.01950000000001,-0.03099999999999,-0.00807716446628533));
#30655=CARTESIAN_POINT('',(0.0120208152801713,-0.03,-0.0155563491861041));
#30656=CARTESIAN_POINT('',(0.0120208152801813,-0.03099999999999,-0.0155563491861141));
#30657=CARTESIAN_POINT('',(0.015556349186104,-0.03,-0.0120208152801713));
#30658=CARTESIAN_POINT('',(0.0109328733497165,-0.02999999999999,-0.0166442911165789));
#30659=CARTESIAN_POINT('',(0.015556349186104,-0.031,-0.0120208152801713));
#30660=CARTESIAN_POINT('',(0.0155563491861141,-0.03099999999999,-0.0120208152801813));
#30661=CARTESIAN_POINT('',(0.01950000000001,-0.03099999999999,-0.00807716446628533));
#30662=CARTESIAN_POINT('Origin',(0.0195,-0.024,-0.008));
#30663=CARTESIAN_POINT('',(0.02087500000001,-0.03099999999999,-0.00800000000000997));
#30664=CARTESIAN_POINT('',(0.0210006091729909,-0.0329651005032875,-0.00800000000000997));
#30665=CARTESIAN_POINT('Origin',(0.025,-0.03275,0.00775));
#30666=CARTESIAN_POINT('',(0.02475000000001,-0.033,0.00775000000001004));
#30667=CARTESIAN_POINT('',(0.02500000000001,-0.03274999999999,0.00775000000001004));
#30668=CARTESIAN_POINT('Origin',(0.02475,-0.03275,-0.008));
#30669=CARTESIAN_POINT('',(0.025,-0.03275,-0.00775));
#30670=CARTESIAN_POINT('',(0.02500000000001,-0.03274999999999,-0.00775000000000996));
#30671=CARTESIAN_POINT('',(0.02475000000001,-0.033,-0.00775000000000996));
#30672=CARTESIAN_POINT('Origin',(0.024875,-0.0328771628421105,-0.007875));
#30673=CARTESIAN_POINT('',(0.025,-0.031,-0.00775));
#30674=CARTESIAN_POINT('',(0.0206250000000099,-0.03099999999999,-0.01212500000001));
#30675=CARTESIAN_POINT('',(0.02500000000001,-0.0328771628421006,-0.00775000000000996));
#30676=CARTESIAN_POINT('Origin',(0.024875,-0.032875,0.004));
#30677=CARTESIAN_POINT('',(0.02500000000001,-0.03274999999999,0.00400000000001004));
#30678=CARTESIAN_POINT('Origin',(0.0105,-0.032875,0.007875));
#30679=CARTESIAN_POINT('',(0.021004363766232,-0.03275,0.008));
#30680=CARTESIAN_POINT('',(0.0105000000000099,-0.03274999999999,0.00800000000001002));
#30681=CARTESIAN_POINT('',(0.0210043631016093,-0.0327500380762109,0.00799996192378913));
#30682=CARTESIAN_POINT('',(0.0208966674520598,-0.0389199177072798,0.00183008229274029));
#30683=CARTESIAN_POINT('',(0.01644626929095,-0.0372292643889901,0.00352073561102997));
#30684=CARTESIAN_POINT('Origin',(0.0175,-0.031,-0.0065));
#30685=CARTESIAN_POINT('',(0.0175,-0.0328,-0.007));
#30686=CARTESIAN_POINT('',(0.017,-0.0328,-0.0065));
#30687=CARTESIAN_POINT('Origin',(0.01750000000001,-0.03279999999999,-0.00650000000000997));
#30688=CARTESIAN_POINT('',(0.0175,-0.031,-0.007));
#30689=CARTESIAN_POINT('',(0.01750000000001,-0.03099999999999,-0.00700000000000997));
#30690=CARTESIAN_POINT('',(0.017,-0.031,-0.0065));
#30691=CARTESIAN_POINT('Origin',(0.01750000000001,-0.03099999999999,-0.00650000000000997));
#30692=CARTESIAN_POINT('',(0.01700000000001,-0.03099999999999,-0.00650000000000997));
#30693=CARTESIAN_POINT('Origin',(0.017,-0.031,-0.007));
#30694=CARTESIAN_POINT('',(0.0235,-0.0328,-0.007));
#30695=CARTESIAN_POINT('',(0.02400000000001,-0.03279999999999,-0.00700000000000996));
#30696=CARTESIAN_POINT('',(0.0235,-0.031,-0.007));
#30697=CARTESIAN_POINT('',(0.02350000000001,-0.03099999999999,-0.00700000000000996));
#30698=CARTESIAN_POINT('',(0.00850000000000998,-0.03099999999999,-0.00700000000000999));
#30699=CARTESIAN_POINT('Origin',(0.0235,-0.031,-0.0065));
#30700=CARTESIAN_POINT('',(0.024,-0.0328,-0.0065));
#30701=CARTESIAN_POINT('Origin',(0.02350000000001,-0.03279999999999,-0.00650000000000996));
#30702=CARTESIAN_POINT('',(0.024,-0.031,-0.0065));
#30703=CARTESIAN_POINT('',(0.02400000000001,-0.03099999999999,-0.00650000000000996));
#30704=CARTESIAN_POINT('Origin',(0.02350000000001,-0.03099999999999,-0.00650000000000996));
#30705=CARTESIAN_POINT('Origin',(0.024,-0.031,-0.007));
#30706=CARTESIAN_POINT('',(0.024,-0.0328,0.0065));
#30707=CARTESIAN_POINT('',(0.02400000000001,-0.03279999999999,0.00700000000001004));
#30708=CARTESIAN_POINT('',(0.024,-0.031,0.0065));
#30709=CARTESIAN_POINT('',(0.02400000000001,-0.03099999999999,0.00650000000001004));
#30710=CARTESIAN_POINT('',(0.02400000000001,-0.03099999999999,-0.00350000000000997));
#30711=CARTESIAN_POINT('Origin',(0.0235,-0.031,0.0065));
#30712=CARTESIAN_POINT('',(0.0235,-0.0328,0.007));
#30713=CARTESIAN_POINT('Origin',(0.02350000000001,-0.03279999999999,0.00650000000001004));
#30714=CARTESIAN_POINT('',(0.0235,-0.031,0.007));
#30715=CARTESIAN_POINT('',(0.02350000000001,-0.03099999999999,0.00700000000001004));
#30716=CARTESIAN_POINT('Origin',(0.02350000000001,-0.03099999999999,0.00650000000001004));
#30717=CARTESIAN_POINT('Origin',(0.024,-0.031,0.007));
#30718=CARTESIAN_POINT('',(0.0175,-0.0328,0.007));
#30719=CARTESIAN_POINT('',(0.01700000000001,-0.03279999999999,0.00700000000001003));
#30720=CARTESIAN_POINT('',(0.0175,-0.031,0.007));
#30721=CARTESIAN_POINT('',(0.01750000000001,-0.03099999999999,0.00700000000001003));
#30722=CARTESIAN_POINT('',(0.0120000000000099,-0.03099999999999,0.00700000000001002));
#30723=CARTESIAN_POINT('Origin',(0.0175,-0.031,0.0065));
#30724=CARTESIAN_POINT('',(0.017,-0.0328,0.0065));
#30725=CARTESIAN_POINT('Origin',(0.01750000000001,-0.03279999999999,0.00650000000001003));
#30726=CARTESIAN_POINT('',(0.017,-0.031,0.0065));
#30727=CARTESIAN_POINT('',(0.01700000000001,-0.03099999999999,0.00650000000001003));
#30728=CARTESIAN_POINT('Origin',(0.01750000000001,-0.03099999999999,0.00650000000001003));
#30729=CARTESIAN_POINT('Origin',(0.0205,-0.0328,3.1147575558204E-17));
#30730=CARTESIAN_POINT('',(0.01700000000001,-0.03279999999999,-0.00700000000000997));
#30731=CARTESIAN_POINT('Origin',(0.017,-0.031,0.007));
#30732=CARTESIAN_POINT('',(0.01700000000001,-0.03099999999999,0.00350000000001003));
#30733=CARTESIAN_POINT('Origin',(0.021,-0.033,-0.016));
#30734=CARTESIAN_POINT('Origin',(0.0208771815508047,-0.0328750190381054,
-0.008));
#30735=CARTESIAN_POINT('',(0.0210043631016192,-0.0327500380762009,-0.00800000000000997));
#30736=CARTESIAN_POINT('Origin',(-4.84735884755548E-17,0.0276710931871507,
3.96791680405306E-31));
#30737=CARTESIAN_POINT('',(-0.00450000000000004,-0.03199999999999,-7.38836374312403E-18));
#30738=CARTESIAN_POINT('Origin',(-4.48806462545766E-17,-0.03199999999999,
3.98348664369065E-31));
#30739=CARTESIAN_POINT('',(-0.00450000000000005,0.0276710931871507,-7.38836374312403E-18));
#30740=CARTESIAN_POINT('Origin',(0.021,-0.033,0.008));
#30741=CARTESIAN_POINT('',(0.0216250000000099,-0.03099999999999,0.00800000000001003));
#30742=CARTESIAN_POINT('',(0.02100000000001,-0.033,0.00800000000001003));
#30743=CARTESIAN_POINT('Origin',(0.025,-0.033,0.008));
#30744=CARTESIAN_POINT('',(0.02500000000001,-0.03099999999999,0.00400000000001004));
#30745=CARTESIAN_POINT('Origin',(0.0155,-0.031,0.0155));
#30746=CARTESIAN_POINT('',(0.0120208152801712,-0.031,0.0155563491861041));
#30747=CARTESIAN_POINT('',(0.015556349186104,-0.031,0.0120208152801713));
#30748=CARTESIAN_POINT('Origin',(0.01550000000001,-0.03099999999999,0.01550000000001));
#30749=CARTESIAN_POINT('',(0.0120208152801712,-0.03,0.0155563491861041));
#30750=CARTESIAN_POINT('',(0.0120208152801812,-0.03099999999999,0.0155563491861141));
#30751=CARTESIAN_POINT('',(0.015556349186104,-0.03,0.0120208152801713));
#30752=CARTESIAN_POINT('Origin',(0.01550000000001,-0.02999999999999,0.01550000000001));
#30753=CARTESIAN_POINT('',(0.0155563491861141,-0.03099999999999,0.0120208152801813));
#30754=CARTESIAN_POINT('Origin',(0.0137883540889866,-0.03,0.0137883540889867));
#30755=CARTESIAN_POINT('',(0.0166442911165788,-0.02999999999999,0.0109328733497165));
#30756=CARTESIAN_POINT('Origin',(0.0155,-0.031,-0.0155));
#30757=CARTESIAN_POINT('Origin',(0.01550000000001,-0.03099999999999,-0.01550000000001));
#30758=CARTESIAN_POINT('Origin',(0.01550000000001,-0.02999999999999,-0.01550000000001));
#30759=CARTESIAN_POINT('Origin',(0.0137883540889867,-0.03,-0.0137883540889867));
#30760=CARTESIAN_POINT('Origin',(-0.0155,-0.031,-0.0155));
#30761=CARTESIAN_POINT('',(-0.0120208152801713,-0.031,-0.0155563491861041));
#30762=CARTESIAN_POINT('',(-0.0155563491861042,-0.031,-0.0120208152801713));
#30763=CARTESIAN_POINT('Origin',(-0.01550000000001,-0.03099999999999,-0.01550000000001));
#30764=CARTESIAN_POINT('',(-0.0120208152801713,-0.03,-0.0155563491861041));
#30765=CARTESIAN_POINT('',(-0.0120208152801813,-0.03099999999999,-0.0155563491861141));
#30766=CARTESIAN_POINT('',(-0.0155563491861042,-0.03,-0.0120208152801713));
#30767=CARTESIAN_POINT('Origin',(-0.01550000000001,-0.02999999999999,-0.01550000000001));
#30768=CARTESIAN_POINT('',(-0.0155563491861142,-0.03099999999999,-0.0120208152801813));
#30769=CARTESIAN_POINT('Origin',(-0.0137883540889867,-0.03,-0.0137883540889867));
#30770=CARTESIAN_POINT('',(-0.0166442911165788,-0.02999999999999,-0.0109328733497165));
#30771=CARTESIAN_POINT('Origin',(0.0195,-0.024,0.00807716446627539));
#30772=CARTESIAN_POINT('',(0.00807716446628528,-0.03099999999999,0.01950000000001));
#30773=CARTESIAN_POINT('',(0.00807716446627529,-0.031,0.0195));
#30774=CARTESIAN_POINT('',(0.00807716446628528,-0.03099999999999,0.01950000000001));
#30775=CARTESIAN_POINT('',(0.00807716446628528,-0.02399999999999,0.01950000000001));
#30776=CARTESIAN_POINT('Origin',(-0.0195,-0.024,-0.00807716446627539));
#30777=CARTESIAN_POINT('',(-0.00807716446627538,-0.031,-0.0195));
#30778=CARTESIAN_POINT('',(-0.00807716446628537,-0.03099999999999,-0.01950000000001));
#30779=CARTESIAN_POINT('',(-0.00807716446628537,-0.02399999999999,-0.01950000000001));
#30780=CARTESIAN_POINT('',(-0.0195,-0.031,-0.00807716446627539));
#30781=CARTESIAN_POINT('',(-0.0195000000000101,-0.02399999999999,-0.00807716446628539));
#30782=CARTESIAN_POINT('',(-0.00807716446628537,-0.03099999999999,-0.01950000000001));
#30783=CARTESIAN_POINT('Origin',(-0.0155,-0.031,0.0155));
#30784=CARTESIAN_POINT('',(-0.0155563491861042,-0.031,0.0120208152801713));
#30785=CARTESIAN_POINT('',(-0.0120208152801714,-0.031,0.0155563491861041));
#30786=CARTESIAN_POINT('Origin',(-0.01550000000001,-0.03099999999999,0.01550000000001));
#30787=CARTESIAN_POINT('',(-0.0155563491861042,-0.03,0.0120208152801713));
#30788=CARTESIAN_POINT('',(-0.0155563491861142,-0.03099999999999,0.0120208152801813));
#30789=CARTESIAN_POINT('',(-0.0120208152801714,-0.03,0.0155563491861041));
#30790=CARTESIAN_POINT('Origin',(-0.01550000000001,-0.02999999999999,0.01550000000001));
#30791=CARTESIAN_POINT('',(-0.0120208152801814,-0.03099999999999,0.0155563491861141));
#30792=CARTESIAN_POINT('Origin',(-0.0137883540889868,-0.03,0.0137883540889867));
#30793=CARTESIAN_POINT('',(-0.0109328733497166,-0.02999999999999,0.0166442911165789));
#30794=CARTESIAN_POINT('Origin',(-0.00807716446627543,-0.024,0.0195));
#30795=CARTESIAN_POINT('',(-0.0195,-0.031,0.00807716446627533));
#30796=CARTESIAN_POINT('',(-0.0195000000000101,-0.03099999999999,0.00807716446628533));
#30797=CARTESIAN_POINT('',(-0.0195000000000101,-0.02399999999999,0.00807716446628533));
#30798=CARTESIAN_POINT('',(-0.00807716446627543,-0.031,0.0195));
#30799=CARTESIAN_POINT('',(-0.00807716446628543,-0.02399999999999,0.01950000000001));
#30800=CARTESIAN_POINT('',(-0.0195000000000101,-0.03099999999999,0.00807716446628533));
#30801=CARTESIAN_POINT('Origin',(0.008,-0.0328750190381054,0.0208771815508047));
#30802=CARTESIAN_POINT('Origin',(-4.54150316748527E-17,-0.023125,3.98117091057093E-31));
#30803=CARTESIAN_POINT('',(0.013,-0.02325,2.13441619245821E-17));
#30804=CARTESIAN_POINT('Origin',(-4.54075051196382E-17,-0.02324999999999,
3.98120352653036E-31));
#30805=CARTESIAN_POINT('',(0.01275,-0.023,2.09336972721863E-17));
#30806=CARTESIAN_POINT('',(0.012875,-0.023125,2.11389295983842E-17));
#30807=CARTESIAN_POINT('Origin',(-4.54225582300685E-17,-0.02299999999999,
3.98113829461149E-31));
#30808=CARTESIAN_POINT('Origin',(-4.54225582300679E-17,-0.023,3.9811382946115E-31));
#30809=CARTESIAN_POINT('',(0.0082500000000029,-0.0229999999999882,1.15246663104728E-17));
#30810=CARTESIAN_POINT('Origin',(-4.54225582300685E-17,-0.02299999999999,
3.98113829461149E-31));
#30811=CARTESIAN_POINT('Origin',(-4.53623457883466E-17,-0.024,3.98139922228696E-31));
#30812=CARTESIAN_POINT('',(0.013,-0.03099999999999,2.13441619245821E-17));
#30813=CARTESIAN_POINT('Origin',(-4.49408586962979E-17,-0.03099999999999,
3.98322571601518E-31));
#30814=CARTESIAN_POINT('',(0.013,-0.024,2.13441619245821E-17));
#30815=CARTESIAN_POINT('Origin',(-4.53924520092072E-17,-0.0235,3.98126875844923E-31));
#30816=CARTESIAN_POINT('',(-0.00800000000001005,-0.02399999999999,-1.21551514373626E-17));
#30817=CARTESIAN_POINT('',(0.0080000000000029,-0.0239999999999882,1.11754339980344E-17));
#30818=CARTESIAN_POINT('Origin',(-4.53623457883472E-17,-0.02399999999999,
3.98139922228695E-31));
#30819=CARTESIAN_POINT('',(0.00812499999999996,-0.0235,1.13500501542495E-17));
#30820=CARTESIAN_POINT('Origin',(-4.53623457883472E-17,-0.02399999999999,
3.98139922228695E-31));
#30821=CARTESIAN_POINT('Origin',(-4.54225582300679E-17,-0.023,3.9811382946115E-31));
#30822=CARTESIAN_POINT('',(-0.00800000000000005,-0.03124999999999,-1.31348688766652E-17));
#30823=CARTESIAN_POINT('',(-0.00800000000000005,-0.023,-1.31348688766652E-17));
#30824=CARTESIAN_POINT('Origin',(-4.49258055858676E-17,-0.03124999999999,
3.98329094793405E-31));
#30825=CARTESIAN_POINT('Origin',(0.0155,-0.0305,-0.0155));
#30826=CARTESIAN_POINT('',(0.0138,-0.03049999999999,-0.0155));
#30827=CARTESIAN_POINT('Origin',(0.01550000000001,-0.03049999999999,-0.01550000000001));
#30828=CARTESIAN_POINT('Origin',(0.0155,0.0276710931871507,-0.0155));
#30829=CARTESIAN_POINT('',(0.0138,0.0276710931871507,-0.0155));
#30830=CARTESIAN_POINT('Origin',(-0.0155,-0.0305,0.0155));
#30831=CARTESIAN_POINT('',(-0.0172,-0.03049999999999,0.0155));
#30832=CARTESIAN_POINT('Origin',(-0.01550000000001,-0.03049999999999,0.01550000000001));
#30833=CARTESIAN_POINT('Origin',(-0.0155,0.0276710931871507,0.0155));
#30834=CARTESIAN_POINT('',(-0.0172,0.0276710931871507,0.0155));
#30835=CARTESIAN_POINT('Origin',(0.0155,-0.0305,0.0155));
#30836=CARTESIAN_POINT('',(0.0138,-0.03049999999999,0.0155));
#30837=CARTESIAN_POINT('Origin',(0.01550000000001,-0.03049999999999,0.01550000000001));
#30838=CARTESIAN_POINT('Origin',(0.0155,0.0276710931871507,0.0155));
#30839=CARTESIAN_POINT('',(0.0138,0.0276710931871507,0.0155));
#30840=CARTESIAN_POINT('Origin',(-0.0155,-0.0305,-0.0155));
#30841=CARTESIAN_POINT('',(-0.0172,-0.03049999999999,-0.0155));
#30842=CARTESIAN_POINT('Origin',(-0.01550000000001,-0.03049999999999,-0.01550000000001));
#30843=CARTESIAN_POINT('Origin',(-0.0155,0.0276710931871507,-0.0155));
#30844=CARTESIAN_POINT('',(-0.0172,0.0276710931871507,-0.0155));
#30845=CARTESIAN_POINT('Origin',(-4.16101896224218E-17,-0.031,1.11022302462556E-18));
#30846=CARTESIAN_POINT('',(0.00807716446628534,-0.03099999999999,-0.01950000000001));
#30847=CARTESIAN_POINT('',(-0.0195000000000101,-0.03099999999999,-0.00807716446628539));
#30848=CARTESIAN_POINT('',(-0.00807716446628543,-0.03099999999999,0.01950000000001));
#30849=CARTESIAN_POINT('Origin',(-4.4925805585867E-17,-0.03125,3.98329094793406E-31));
#30850=CARTESIAN_POINT('',(-0.00600000000000004,-0.03124999999999,-9.85115165749883E-18));
#30851=CARTESIAN_POINT('Origin',(-4.49258055858676E-17,-0.03124999999999,
3.98329094793405E-31));
#30852=CARTESIAN_POINT('',(-0.00600000000000004,-0.03199999999999,-9.85115165749883E-18));
#30853=CARTESIAN_POINT('',(-0.00600000000000004,-0.03125,-9.85115165749883E-18));
#30854=CARTESIAN_POINT('Origin',(-4.48806462545766E-17,-0.03199999999999,
3.98348664369065E-31));
#30855=CARTESIAN_POINT('Origin',(-4.4880646254576E-17,-0.032,3.98348664369065E-31));
#30856=CARTESIAN_POINT('Origin',(-4.4925805585867E-17,-0.03125,3.98329094793406E-31));
#30857=CARTESIAN_POINT('Origin',(-0.00807716446627538,-0.024,-0.0195));
#30858=CARTESIAN_POINT('Origin',(-0.0195,-0.024,0.00807716446627533));
#30859=CARTESIAN_POINT('Origin',(0.00807716446627529,-0.024,0.0195));
#30860=CARTESIAN_POINT('Origin',(0.021,-0.033,-0.016));
#34813=UNCERTAINTY_MEASURE_WITH_UNIT(LENGTH_MEASURE(1.E-5),#34877,
'DISTANCE_ACCURACY_VALUE',
'Maximum model space distance between geometric entities at asserted c
onnectivities');
#34841=UNCERTAINTY_MEASURE_WITH_UNIT(LENGTH_MEASURE(1.E-5),#34877,
'DISTANCE_ACCURACY_VALUE',
'Maximum model space distance between geometric entities at asserted c
onnectivities');
#34848=(
GEOMETRIC_REPRESENTATION_CONTEXT(3)
GLOBAL_UNCERTAINTY_ASSIGNED_CONTEXT((#34813))
GLOBAL_UNIT_ASSIGNED_CONTEXT((#34877,#34878,#34879))
REPRESENTATION_CONTEXT('','3D')
);
#34876=(
GEOMETRIC_REPRESENTATION_CONTEXT(3)
GLOBAL_UNCERTAINTY_ASSIGNED_CONTEXT((#34841))
GLOBAL_UNIT_ASSIGNED_CONTEXT((#34877,#34878,#34879))
REPRESENTATION_CONTEXT('','3D')
);
#34877=(
LENGTH_UNIT()
NAMED_UNIT(*)
SI_UNIT($,.METRE.)
);
#34878=(
NAMED_UNIT(*)
PLANE_ANGLE_UNIT()
SI_UNIT($,.RADIAN.)
);
#34879=(
NAMED_UNIT(*)
SI_UNIT($,.STERADIAN.)
SOLID_ANGLE_UNIT()
);
#34886=SHAPE_DEFINITION_REPRESENTATION(#34920,#34990);
#34920=PRODUCT_DEFINITION_SHAPE('',$,#35025);
#34990=SHAPE_REPRESENTATION('',(#20591),#34848);
#35018=PRODUCT_DEFINITION_CONTEXT('part definition',#35122,'design');
#35025=PRODUCT_DEFINITION('Motor Base Cap','Motor Base Cap',#35059,#35018);
#35059=PRODUCT_DEFINITION_FORMATION('',$,#35130);
#35122=APPLICATION_CONTEXT('Managed model based 3d engineering');
#35123=PRODUCT_CONTEXT('part definition',#35122,'mechanical');
#35130=PRODUCT('Motor Base Cap','Motor Base Cap',
'LEGAL AND USAGE DISCLAIMER: this Data/Model is provided \X2\201C\X0\A
S IS\X2\201D\X0\ for informational and representational only. It is a 
geometric approximation and is NOT engineered, certified, or guarantee
d for dimensional accuracy, exact tolerances, or production-level prec
ision. Vendor disclaims all implied warranties including fitness for a
 particular purpose. DO NOT USE FOR DIRECT PHYSICAL MANUFACTURING, AUT
OMATED PRODUCTION, OR SAFETY-CRITICAL SYSTEMS without independent engi
neering verification and resolution of any design discrepancies.',(#35123));
#35159=PRESENTATION_STYLE_ASSIGNMENT((#35168));
#35168=SURFACE_STYLE_USAGE(.BOTH.,#35177);
#35177=SURFACE_SIDE_STYLE('',(#35186));
#35186=SURFACE_STYLE_FILL_AREA(#35195);
#35195=FILL_AREA_STYLE('Paint - Enamel Glossy (White)',(#35204));
#35204=FILL_AREA_STYLE_COLOUR('Paint - Enamel Glossy (White)',#35213);
#35213=COLOUR_RGB('Paint - Enamel Glossy (White)',0.964705882352941,0.964705882352941,
0.952941176470588);
ENDSEC;
END-ISO-10303-21;
